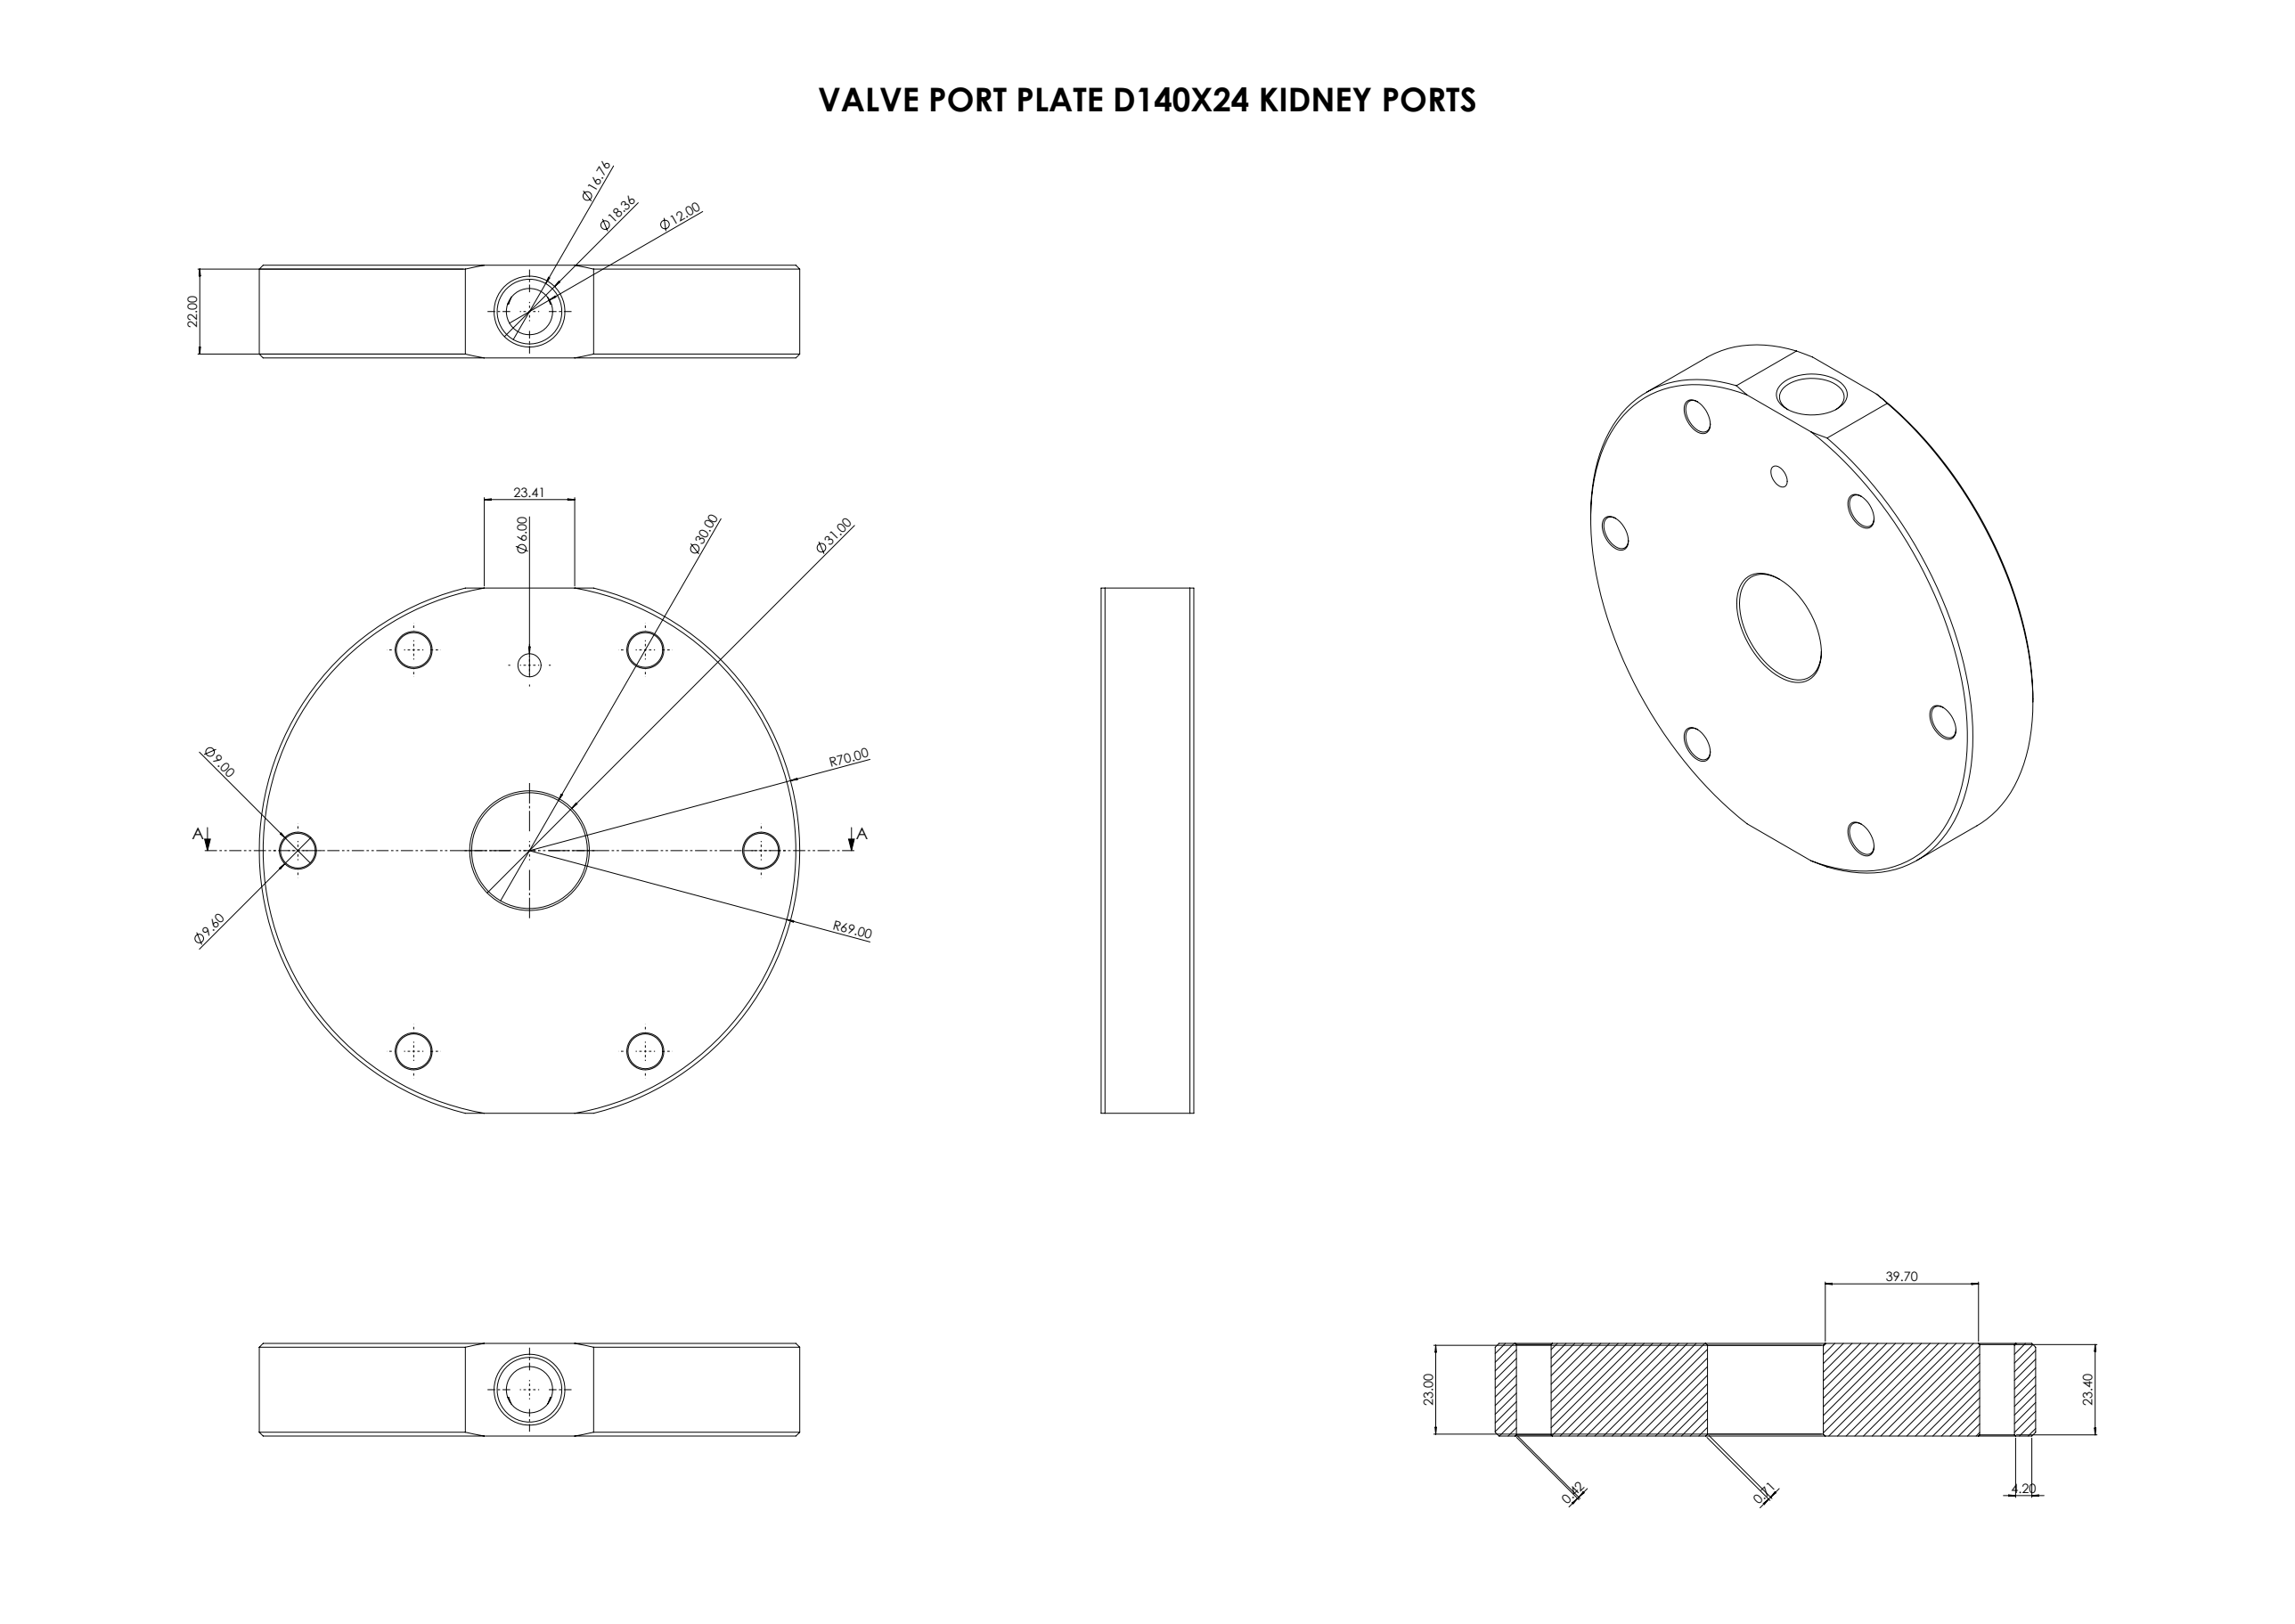
ISO-10303-21;
HEADER;
/* Generated by software containing ST-Developer
 * from STEP Tools, Inc. (www.steptools.com) 
 */

FILE_DESCRIPTION(
/* description */ (''),
/* implementation_level */ '2;1');

FILE_NAME(
/* name */ '02_Valve_Port_Plate_D140x24_Kidney_Ports.step',
/* time_stamp */ '2026-10-23T00:52:27+05:00',
/* author */ (''),
/* organization */ (''),
/* preprocessor_version */ 'ST-DEVELOPER v20.2',
/* originating_system */ 'Autodesk Translation Framework v15.15.0.0',
/* authorisation */ '');

FILE_SCHEMA (('AUTOMOTIVE_DESIGN { 1 0 10303 214 3 1 1 }'));
ENDSEC;

DATA;
#10=MECHANICAL_DESIGN_GEOMETRIC_PRESENTATION_REPRESENTATION('',(#1565),#59204);
#704=B_SPLINE_CURVE_WITH_KNOTS('',3,(#42904,#42905,#42906,#42907,#42908,
#42909,#42910,#42911,#42912,#42913,#42914,#42915,#42916,#42917,#42918,#42919,
#42920,#42921),.UNSPECIFIED.,.F.,.F.,(4,2,2,2,2,2,2,2,4),(0.,0.115474560264442,
0.230949120528883,0.346108891526704,0.461268662524524,0.576428433522344,
0.691588204520164,0.807062764784606,0.922537325049047),.UNSPECIFIED.);
#705=B_SPLINE_CURVE_WITH_KNOTS('',3,(#42922,#42923,#42924,#42925,#42926,
#42927,#42928,#42929,#42930,#42931,#42932,#42933,#42934,#42935,#42936,#42937,
#42938,#42939),.UNSPECIFIED.,.F.,.F.,(4,2,2,2,2,2,2,2,4),(0.922537325049047,
1.03801188531349,1.15348644557793,1.26864621657575,1.38380598757357,1.49896575857139,
1.61412552956921,1.72960008983365,1.84507465009809),.UNSPECIFIED.);
#706=B_SPLINE_CURVE_WITH_KNOTS('',3,(#43005,#43006,#43007,#43008,#43009,
#43010,#43011,#43012,#43013,#43014),.UNSPECIFIED.,.F.,.F.,(4,2,2,2,4),(0.196434861767707,
0.226700589297083,0.453401178594166,0.680088163565136,0.906775148536106),
 .UNSPECIFIED.);
#707=B_SPLINE_CURVE_WITH_KNOTS('',3,(#43021,#43022,#43023,#43024,#43025,
#43026,#43027,#43028,#43029,#43030),.UNSPECIFIED.,.F.,.F.,(4,2,2,2,4),(0.906775148536106,
1.13346213350708,1.36014911847805,1.58684970777513,1.61711543530451),
 .UNSPECIFIED.);
#708=B_SPLINE_CURVE_WITH_KNOTS('',3,(#43034,#43035,#43036,#43037,#43038,
#43039,#43040,#43041,#43042,#43043,#43044,#43045,#43046,#43047),
 .UNSPECIFIED.,.F.,.F.,(4,2,2,2,2,2,4),(2.20122847938268,2.27205851753461,
2.49923948385036,2.72642045016611,2.95360141648186,3.18078238279761,3.25161242094954),
 .UNSPECIFIED.);
#709=B_SPLINE_CURVE_WITH_KNOTS('',3,(#43054,#43055,#43056,#43057,#43058,
#43059),.UNSPECIFIED.,.F.,.F.,(4,2,4),(0.193270693145506,0.23055183180291,
0.366122014076097),.UNSPECIFIED.);
#710=B_SPLINE_CURVE_WITH_KNOTS('',3,(#43067,#43068,#43069,#43070,#43071,
#43072),.UNSPECIFIED.,.F.,.F.,(4,2,4),(1.5242057805381,1.65977596281129,
1.69705710146869),.UNSPECIFIED.);
#711=B_SPLINE_CURVE_WITH_KNOTS('',3,(#43096,#43097,#43098,#43099,#43100,
#43101,#43102,#43103,#43104,#43105),.UNSPECIFIED.,.F.,.F.,(4,2,2,2,4),(2.72032544560832,
2.94701243057929,3.17369941555026,3.40040000484734,3.43066573237672),
 .UNSPECIFIED.);
#712=B_SPLINE_CURVE_WITH_KNOTS('',3,(#43110,#43111,#43112,#43113,#43114,
#43115,#43116,#43117,#43118,#43119),.UNSPECIFIED.,.F.,.F.,(4,2,2,2,4),(2.00998515883992,
2.0402508863693,2.26695147566638,2.49363846063735,2.72032544560832),
 .UNSPECIFIED.);
#713=B_SPLINE_CURVE_WITH_KNOTS('',3,(#43126,#43127,#43128,#43129,#43130,
#43131,#43132,#43133,#43134,#43135,#43136,#43137,#43138,#43139),
 .UNSPECIFIED.,.F.,.F.,(4,2,2,2,2,2,4),(0.383614845938606,0.454444884090536,
0.681625850406286,0.908806816722037,1.13598778303779,1.36316874935354,1.43399878750547),
 .UNSPECIFIED.);
#714=B_SPLINE_CURVE_WITH_KNOTS('',3,(#43147,#43148,#43149,#43150,#43151,
#43152),.UNSPECIFIED.,.F.,.F.,(4,2,4),(2.08359848775971,2.12087962641711,
2.2564498086903),.UNSPECIFIED.);
#715=B_SPLINE_CURVE_WITH_KNOTS('',3,(#43160,#43161,#43162,#43163,#43164,
#43165),.UNSPECIFIED.,.F.,.F.,(4,2,4),(3.4145335751523,3.55010375742549,
3.5873848960829),.UNSPECIFIED.);
#1482=(
BOUNDED_CURVE()
B_SPLINE_CURVE(2,(#42953,#42954,#42955),.UNSPECIFIED.,.F.,.F.)
B_SPLINE_CURVE_WITH_KNOTS((3,3),(0.,0.501003712116266),.UNSPECIFIED.)
CURVE()
GEOMETRIC_REPRESENTATION_ITEM()
RATIONAL_B_SPLINE_CURVE((1.,1.00062409811598,1.))
REPRESENTATION_ITEM('')
);
#1483=(
BOUNDED_CURVE()
B_SPLINE_CURVE(2,(#42958,#42959,#42960),.UNSPECIFIED.,.F.,.F.)
B_SPLINE_CURVE_WITH_KNOTS((3,3),(0.,0.501003712116271),.UNSPECIFIED.)
CURVE()
GEOMETRIC_REPRESENTATION_ITEM()
RATIONAL_B_SPLINE_CURVE((1.,1.00062409811548,1.))
REPRESENTATION_ITEM('')
);
#1484=(
BOUNDED_CURVE()
B_SPLINE_CURVE(2,(#42962,#42963,#42964),.UNSPECIFIED.,.F.,.F.)
B_SPLINE_CURVE_WITH_KNOTS((3,3),(0.,0.501003712116271),.UNSPECIFIED.)
CURVE()
GEOMETRIC_REPRESENTATION_ITEM()
RATIONAL_B_SPLINE_CURVE((1.,1.00062409811548,1.))
REPRESENTATION_ITEM('')
);
#1485=(
BOUNDED_CURVE()
B_SPLINE_CURVE(2,(#42967,#42968,#42969),.UNSPECIFIED.,.F.,.F.)
B_SPLINE_CURVE_WITH_KNOTS((3,3),(0.,0.501003712116266),.UNSPECIFIED.)
CURVE()
GEOMETRIC_REPRESENTATION_ITEM()
RATIONAL_B_SPLINE_CURVE((1.,1.00062409811598,1.))
REPRESENTATION_ITEM('')
);
#1486=(
BOUNDED_CURVE()
B_SPLINE_CURVE(2,(#42982,#42983,#42984),.UNSPECIFIED.,.F.,.F.)
B_SPLINE_CURVE_WITH_KNOTS((3,3),(0.,0.501003712116266),.UNSPECIFIED.)
CURVE()
GEOMETRIC_REPRESENTATION_ITEM()
RATIONAL_B_SPLINE_CURVE((1.,1.00062409811598,1.))
REPRESENTATION_ITEM('')
);
#1487=(
BOUNDED_CURVE()
B_SPLINE_CURVE(2,(#42987,#42988,#42989),.UNSPECIFIED.,.F.,.F.)
B_SPLINE_CURVE_WITH_KNOTS((3,3),(0.,0.501003712116271),.UNSPECIFIED.)
CURVE()
GEOMETRIC_REPRESENTATION_ITEM()
RATIONAL_B_SPLINE_CURVE((1.,1.00062409811541,1.))
REPRESENTATION_ITEM('')
);
#1488=(
BOUNDED_CURVE()
B_SPLINE_CURVE(2,(#42991,#42992,#42993),.UNSPECIFIED.,.F.,.F.)
B_SPLINE_CURVE_WITH_KNOTS((3,3),(0.,0.501003712116271),.UNSPECIFIED.)
CURVE()
GEOMETRIC_REPRESENTATION_ITEM()
RATIONAL_B_SPLINE_CURVE((1.,1.00062409811541,1.))
REPRESENTATION_ITEM('')
);
#1489=(
BOUNDED_CURVE()
B_SPLINE_CURVE(2,(#42996,#42997,#42998),.UNSPECIFIED.,.F.,.F.)
B_SPLINE_CURVE_WITH_KNOTS((3,3),(0.,0.501003712116266),.UNSPECIFIED.)
CURVE()
GEOMETRIC_REPRESENTATION_ITEM()
RATIONAL_B_SPLINE_CURVE((1.,1.00062409811598,1.))
REPRESENTATION_ITEM('')
);
#1490=(
BOUNDED_CURVE()
B_SPLINE_CURVE(2,(#43060,#43061,#43062),.UNSPECIFIED.,.F.,.F.)
B_SPLINE_CURVE_WITH_KNOTS((3,3),(0.,0.0102434961117393),.UNSPECIFIED.)
CURVE()
GEOMETRIC_REPRESENTATION_ITEM()
RATIONAL_B_SPLINE_CURVE((1.,1.01666622123361,1.03305467953702))
REPRESENTATION_ITEM('')
);
#1491=(
BOUNDED_CURVE()
B_SPLINE_CURVE(2,(#43064,#43065,#43066),.UNSPECIFIED.,.F.,.F.)
B_SPLINE_CURVE_WITH_KNOTS((3,3),(1.21900889027555,1.22925238638729),
 .UNSPECIFIED.)
CURVE()
GEOMETRIC_REPRESENTATION_ITEM()
RATIONAL_B_SPLINE_CURVE((1.03305467953703,1.01666622123362,1.))
REPRESENTATION_ITEM('')
);
#1492=(
BOUNDED_CURVE()
B_SPLINE_CURVE(2,(#43153,#43154,#43155),.UNSPECIFIED.,.F.,.F.)
B_SPLINE_CURVE_WITH_KNOTS((3,3),(0.,0.0102434961117392),.UNSPECIFIED.)
CURVE()
GEOMETRIC_REPRESENTATION_ITEM()
RATIONAL_B_SPLINE_CURVE((1.,1.01666622123361,1.03305467953702))
REPRESENTATION_ITEM('')
);
#1493=(
BOUNDED_CURVE()
B_SPLINE_CURVE(2,(#43157,#43158,#43159),.UNSPECIFIED.,.F.,.F.)
B_SPLINE_CURVE_WITH_KNOTS((3,3),(1.21900889027555,1.22925238638729),
 .UNSPECIFIED.)
CURVE()
GEOMETRIC_REPRESENTATION_ITEM()
RATIONAL_B_SPLINE_CURVE((1.03305467953701,1.01666622123361,1.))
REPRESENTATION_ITEM('')
);
#1519=SHAPE_REPRESENTATION_RELATIONSHIP('SRR','None',#59308,#1539);
#1539=ADVANCED_BREP_SHAPE_REPRESENTATION('',(#1586),#59195);
#1565=STYLED_ITEM('',(#59579),#1586);
#1586=MANIFOLD_SOLID_BREP('Valve plate',#22815);
#1694=FACE_BOUND('',#4510,.T.);
#1695=FACE_BOUND('',#4511,.T.);
#1696=FACE_BOUND('',#4512,.T.);
#1697=FACE_BOUND('',#4513,.T.);
#1698=FACE_BOUND('',#4514,.T.);
#1699=FACE_BOUND('',#4515,.T.);
#1700=FACE_BOUND('',#4516,.T.);
#1701=FACE_BOUND('',#4517,.T.);
#1702=FACE_BOUND('',#4520,.T.);
#1703=FACE_BOUND('',#4521,.T.);
#1704=FACE_BOUND('',#4522,.T.);
#1705=FACE_BOUND('',#4523,.T.);
#1706=FACE_BOUND('',#4524,.T.);
#1707=FACE_BOUND('',#4525,.T.);
#1708=FACE_BOUND('',#4526,.T.);
#1709=FACE_BOUND('',#4527,.T.);
#1710=FACE_BOUND('',#4528,.T.);
#1711=FACE_BOUND('',#4548,.T.);
#1712=FACE_BOUND('',#4552,.T.);
#1713=FACE_BOUND('',#4556,.T.);
#1714=FACE_BOUND('',#4564,.T.);
#1715=FACE_BOUND('',#4568,.T.);
#2041=PLANE('',#23872);
#2042=PLANE('',#23884);
#2043=PLANE('',#23932);
#2044=PLANE('',#23938);
#2045=PLANE('',#23945);
#2046=PLANE('',#23950);
#2047=PLANE('',#23965);
#2048=PLANE('',#23969);
#2049=PLANE('',#23977);
#2050=PLANE('',#23983);
#2529=CYLINDRICAL_SURFACE('',#23870,0.45);
#2530=CYLINDRICAL_SURFACE('',#23903,0.45);
#2531=CYLINDRICAL_SURFACE('',#23908,0.45);
#2532=CYLINDRICAL_SURFACE('',#23913,0.45);
#2533=CYLINDRICAL_SURFACE('',#23918,0.45);
#2534=CYLINDRICAL_SURFACE('',#23923,0.45);
#2535=CYLINDRICAL_SURFACE('',#23926,0.3);
#2536=CYLINDRICAL_SURFACE('',#23930,0.8381);
#2537=CYLINDRICAL_SURFACE('',#23936,0.8381);
#2538=CYLINDRICAL_SURFACE('',#23939,0.6);
#2539=CYLINDRICAL_SURFACE('',#23942,0.6);
#2540=CYLINDRICAL_SURFACE('',#23947,2.25);
#2541=CYLINDRICAL_SURFACE('',#23955,7.);
#2542=CYLINDRICAL_SURFACE('',#23958,0.6);
#2543=CYLINDRICAL_SURFACE('',#23961,0.6);
#2544=CYLINDRICAL_SURFACE('',#23966,2.25);
#2545=CYLINDRICAL_SURFACE('',#23972,0.35);
#2546=CYLINDRICAL_SURFACE('',#23974,2.95);
#2547=CYLINDRICAL_SURFACE('',#23976,0.35);
#2548=CYLINDRICAL_SURFACE('',#23978,0.35);
#2549=CYLINDRICAL_SURFACE('',#23980,2.95);
#2550=CYLINDRICAL_SURFACE('',#23982,0.35);
#2551=CYLINDRICAL_SURFACE('',#23987,1.5);
#2552=CYLINDRICAL_SURFACE('',#23993,7.);
#3107=FACE_OUTER_BOUND('',#4507,.T.);
#3108=FACE_OUTER_BOUND('',#4508,.T.);
#3109=FACE_OUTER_BOUND('',#4509,.T.);
#3110=FACE_OUTER_BOUND('',#4518,.T.);
#3111=FACE_OUTER_BOUND('',#4519,.T.);
#3112=FACE_OUTER_BOUND('',#4529,.T.);
#3113=FACE_OUTER_BOUND('',#4530,.T.);
#3114=FACE_OUTER_BOUND('',#4531,.T.);
#3115=FACE_OUTER_BOUND('',#4532,.T.);
#3116=FACE_OUTER_BOUND('',#4533,.T.);
#3117=FACE_OUTER_BOUND('',#4534,.T.);
#3118=FACE_OUTER_BOUND('',#4535,.T.);
#3119=FACE_OUTER_BOUND('',#4536,.T.);
#3120=FACE_OUTER_BOUND('',#4537,.T.);
#3121=FACE_OUTER_BOUND('',#4538,.T.);
#3122=FACE_OUTER_BOUND('',#4539,.T.);
#3123=FACE_OUTER_BOUND('',#4540,.T.);
#3124=FACE_OUTER_BOUND('',#4541,.T.);
#3125=FACE_OUTER_BOUND('',#4542,.T.);
#3126=FACE_OUTER_BOUND('',#4543,.T.);
#3127=FACE_OUTER_BOUND('',#4544,.T.);
#3128=FACE_OUTER_BOUND('',#4545,.T.);
#3129=FACE_OUTER_BOUND('',#4546,.T.);
#3130=FACE_OUTER_BOUND('',#4547,.T.);
#3131=FACE_OUTER_BOUND('',#4549,.T.);
#3132=FACE_OUTER_BOUND('',#4550,.T.);
#3133=FACE_OUTER_BOUND('',#4551,.T.);
#3134=FACE_OUTER_BOUND('',#4553,.T.);
#3135=FACE_OUTER_BOUND('',#4554,.T.);
#3136=FACE_OUTER_BOUND('',#4555,.T.);
#3137=FACE_OUTER_BOUND('',#4557,.T.);
#3138=FACE_OUTER_BOUND('',#4558,.T.);
#3139=FACE_OUTER_BOUND('',#4559,.T.);
#3140=FACE_OUTER_BOUND('',#4560,.T.);
#3141=FACE_OUTER_BOUND('',#4561,.T.);
#3142=FACE_OUTER_BOUND('',#4562,.T.);
#3143=FACE_OUTER_BOUND('',#4563,.T.);
#3144=FACE_OUTER_BOUND('',#4565,.T.);
#3145=FACE_OUTER_BOUND('',#4566,.T.);
#3146=FACE_OUTER_BOUND('',#4567,.T.);
#3147=FACE_OUTER_BOUND('',#4569,.T.);
#3148=FACE_OUTER_BOUND('',#4570,.T.);
#3149=FACE_OUTER_BOUND('',#4571,.T.);
#3150=FACE_OUTER_BOUND('',#4572,.T.);
#3151=FACE_OUTER_BOUND('',#4573,.T.);
#3152=FACE_OUTER_BOUND('',#4574,.T.);
#3153=FACE_OUTER_BOUND('',#4575,.T.);
#3154=FACE_OUTER_BOUND('',#4576,.T.);
#3155=FACE_OUTER_BOUND('',#4577,.T.);
#3156=FACE_OUTER_BOUND('',#4578,.T.);
#3157=FACE_OUTER_BOUND('',#4579,.T.);
#3158=FACE_OUTER_BOUND('',#4580,.T.);
#3159=FACE_OUTER_BOUND('',#4581,.T.);
#3160=FACE_OUTER_BOUND('',#4582,.T.);
#3161=FACE_OUTER_BOUND('',#4583,.T.);
#3162=FACE_OUTER_BOUND('',#4584,.T.);
#4507=EDGE_LOOP('',(#16736,#16737,#16738,#16739));
#4508=EDGE_LOOP('',(#16740,#16741,#16742,#16743));
#4509=EDGE_LOOP('',(#16744,#16745,#16746,#16747));
#4510=EDGE_LOOP('',(#16748));
#4511=EDGE_LOOP('',(#16749));
#4512=EDGE_LOOP('',(#16750));
#4513=EDGE_LOOP('',(#16751));
#4514=EDGE_LOOP('',(#16752));
#4515=EDGE_LOOP('',(#16753));
#4516=EDGE_LOOP('',(#16754));
#4517=EDGE_LOOP('',(#16755));
#4518=EDGE_LOOP('',(#16756,#16757,#16758,#16759));
#4519=EDGE_LOOP('',(#16760,#16761,#16762,#16763));
#4520=EDGE_LOOP('',(#16764));
#4521=EDGE_LOOP('',(#16765));
#4522=EDGE_LOOP('',(#16766));
#4523=EDGE_LOOP('',(#16767,#16768,#16769,#16770));
#4524=EDGE_LOOP('',(#16771,#16772,#16773,#16774));
#4525=EDGE_LOOP('',(#16775));
#4526=EDGE_LOOP('',(#16776));
#4527=EDGE_LOOP('',(#16777));
#4528=EDGE_LOOP('',(#16778));
#4529=EDGE_LOOP('',(#16779,#16780,#16781,#16782));
#4530=EDGE_LOOP('',(#16783,#16784,#16785,#16786));
#4531=EDGE_LOOP('',(#16787,#16788,#16789,#16790));
#4532=EDGE_LOOP('',(#16791,#16792,#16793,#16794));
#4533=EDGE_LOOP('',(#16795,#16796,#16797,#16798));
#4534=EDGE_LOOP('',(#16799,#16800,#16801,#16802));
#4535=EDGE_LOOP('',(#16803,#16804,#16805,#16806));
#4536=EDGE_LOOP('',(#16807,#16808,#16809,#16810));
#4537=EDGE_LOOP('',(#16811,#16812,#16813,#16814));
#4538=EDGE_LOOP('',(#16815,#16816,#16817,#16818));
#4539=EDGE_LOOP('',(#16819,#16820,#16821,#16822));
#4540=EDGE_LOOP('',(#16823,#16824,#16825,#16826));
#4541=EDGE_LOOP('',(#16827,#16828,#16829,#16830));
#4542=EDGE_LOOP('',(#16831,#16832,#16833,#16834));
#4543=EDGE_LOOP('',(#16835,#16836,#16837,#16838));
#4544=EDGE_LOOP('',(#16839,#16840,#16841,#16842,#16843));
#4545=EDGE_LOOP('',(#16844,#16845,#16846,#16847));
#4546=EDGE_LOOP('',(#16848,#16849,#16850,#16851));
#4547=EDGE_LOOP('',(#16852,#16853,#16854,#16855,#16856,#16857,#16858,#16859));
#4548=EDGE_LOOP('',(#16860));
#4549=EDGE_LOOP('',(#16861,#16862,#16863,#16864));
#4550=EDGE_LOOP('',(#16865,#16866,#16867,#16868));
#4551=EDGE_LOOP('',(#16869,#16870,#16871,#16872,#16873,#16874,#16875,#16876));
#4552=EDGE_LOOP('',(#16877));
#4553=EDGE_LOOP('',(#16878,#16879,#16880,#16881,#16882,#16883,#16884,#16885));
#4554=EDGE_LOOP('',(#16886,#16887,#16888));
#4555=EDGE_LOOP('',(#16889));
#4556=EDGE_LOOP('',(#16890));
#4557=EDGE_LOOP('',(#16891,#16892,#16893,#16894,#16895,#16896,#16897,#16898,
#16899));
#4558=EDGE_LOOP('',(#16900,#16901,#16902,#16903,#16904,#16905,#16906,#16907));
#4559=EDGE_LOOP('',(#16908,#16909,#16910,#16911,#16912));
#4560=EDGE_LOOP('',(#16913,#16914,#16915,#16916));
#4561=EDGE_LOOP('',(#16917,#16918,#16919,#16920));
#4562=EDGE_LOOP('',(#16921,#16922,#16923,#16924));
#4563=EDGE_LOOP('',(#16925,#16926,#16927,#16928,#16929,#16930,#16931,#16932));
#4564=EDGE_LOOP('',(#16933,#16934));
#4565=EDGE_LOOP('',(#16935,#16936,#16937));
#4566=EDGE_LOOP('',(#16938,#16939,#16940,#16941,#16942,#16943,#16944,#16945,
#16946));
#4567=EDGE_LOOP('',(#16947));
#4568=EDGE_LOOP('',(#16948));
#4569=EDGE_LOOP('',(#16949,#16950,#16951,#16952,#16953,#16954,#16955,#16956));
#4570=EDGE_LOOP('',(#16957,#16958,#16959,#16960,#16961));
#4571=EDGE_LOOP('',(#16962,#16963,#16964,#16965));
#4572=EDGE_LOOP('',(#16966,#16967,#16968,#16969,#16970,#16971,#16972));
#4573=EDGE_LOOP('',(#16973,#16974,#16975,#16976));
#4574=EDGE_LOOP('',(#16977,#16978,#16979,#16980,#16981));
#4575=EDGE_LOOP('',(#16982,#16983,#16984,#16985));
#4576=EDGE_LOOP('',(#16986,#16987,#16988,#16989,#16990,#16991,#16992));
#4577=EDGE_LOOP('',(#16993,#16994,#16995,#16996));
#4578=EDGE_LOOP('',(#16997,#16998,#16999,#17000,#17001));
#4579=EDGE_LOOP('',(#17002,#17003,#17004,#17005,#17006));
#4580=EDGE_LOOP('',(#17007,#17008,#17009,#17010,#17011,#17012));
#4581=EDGE_LOOP('',(#17013,#17014,#17015,#17016,#17017));
#4582=EDGE_LOOP('',(#17018,#17019,#17020,#17021));
#4583=EDGE_LOOP('',(#17022,#17023,#17024,#17025));
#4584=EDGE_LOOP('',(#17026,#17027,#17028,#17029));
#5973=LINE('',#42781,#7406);
#5974=LINE('',#42786,#7407);
#5975=LINE('',#42790,#7408);
#5976=LINE('',#42794,#7409);
#5977=LINE('',#42813,#7410);
#5978=LINE('',#42817,#7411);
#5979=LINE('',#42821,#7412);
#5980=LINE('',#42853,#7413);
#5981=LINE('',#42858,#7414);
#5982=LINE('',#42860,#7415);
#5983=LINE('',#42863,#7416);
#5984=LINE('',#42868,#7417);
#5985=LINE('',#42870,#7418);
#5986=LINE('',#42873,#7419);
#5987=LINE('',#42878,#7420);
#5988=LINE('',#42880,#7421);
#5989=LINE('',#42883,#7422);
#5990=LINE('',#42888,#7423);
#5991=LINE('',#42890,#7424);
#5992=LINE('',#42893,#7425);
#5993=LINE('',#42898,#7426);
#5994=LINE('',#42900,#7427);
#5995=LINE('',#42940,#7428);
#5996=LINE('',#42945,#7429);
#5997=LINE('',#42950,#7430);
#5998=LINE('',#42957,#7431);
#5999=LINE('',#42966,#7432);
#6000=LINE('',#42974,#7433);
#6001=LINE('',#42978,#7434);
#6002=LINE('',#42986,#7435);
#6003=LINE('',#42995,#7436);
#6004=LINE('',#43003,#7437);
#6005=LINE('',#43016,#7438);
#6006=LINE('',#43020,#7439);
#6007=LINE('',#43074,#7440);
#6008=LINE('',#43078,#7441);
#6009=LINE('',#43080,#7442);
#6010=LINE('',#43094,#7443);
#6011=LINE('',#43107,#7444);
#6012=LINE('',#43121,#7445);
#6013=LINE('',#43145,#7446);
#6014=LINE('',#43170,#7447);
#6015=LINE('',#43172,#7448);
#6016=LINE('',#43180,#7449);
#6017=LINE('',#43184,#7450);
#6018=LINE('',#43189,#7451);
#6019=LINE('',#43193,#7452);
#6020=LINE('',#43198,#7453);
#6021=LINE('',#43207,#7454);
#6022=LINE('',#43209,#7455);
#7406=VECTOR('',#27247,0.465);
#7407=VECTOR('',#27254,0.45);
#7408=VECTOR('',#27257,1.);
#7409=VECTOR('',#27260,1.);
#7410=VECTOR('',#27281,0.465);
#7411=VECTOR('',#27284,1.);
#7412=VECTOR('',#27287,1.);
#7413=VECTOR('',#27320,0.465);
#7414=VECTOR('',#27327,0.45);
#7415=VECTOR('',#27330,0.465);
#7416=VECTOR('',#27333,0.465);
#7417=VECTOR('',#27340,0.45);
#7418=VECTOR('',#27343,0.465);
#7419=VECTOR('',#27346,0.465);
#7420=VECTOR('',#27353,0.45);
#7421=VECTOR('',#27356,0.465);
#7422=VECTOR('',#27359,0.465);
#7423=VECTOR('',#27366,0.45);
#7424=VECTOR('',#27369,0.465);
#7425=VECTOR('',#27372,0.465);
#7426=VECTOR('',#27379,0.45);
#7427=VECTOR('',#27382,0.465);
#7428=VECTOR('',#27385,0.3);
#7429=VECTOR('',#27390,0.8781);
#7430=VECTOR('',#27397,0.8381);
#7431=VECTOR('',#27400,1.);
#7432=VECTOR('',#27401,1.);
#7433=VECTOR('',#27406,0.8781);
#7434=VECTOR('',#27411,0.8381);
#7435=VECTOR('',#27416,1.);
#7436=VECTOR('',#27417,1.);
#7437=VECTOR('',#27422,0.6);
#7438=VECTOR('',#27423,1.);
#7439=VECTOR('',#27426,1.);
#7440=VECTOR('',#27437,0.6);
#7441=VECTOR('',#27442,1.);
#7442=VECTOR('',#27443,1.);
#7443=VECTOR('',#27464,1.);
#7444=VECTOR('',#27465,0.6);
#7445=VECTOR('',#27468,1.);
#7446=VECTOR('',#27479,0.3);
#7447=VECTOR('',#27486,1.);
#7448=VECTOR('',#27487,1.);
#7449=VECTOR('',#27498,1.);
#7450=VECTOR('',#27505,1.);
#7451=VECTOR('',#27512,1.);
#7452=VECTOR('',#27519,1.);
#7453=VECTOR('',#27526,1.525);
#7454=VECTOR('',#27537,1.5);
#7455=VECTOR('',#27540,1.525);
#8745=CIRCLE('',#23868,0.48);
#8746=CIRCLE('',#23869,0.45);
#8747=CIRCLE('',#23871,0.45);
#8748=CIRCLE('',#23873,6.9);
#8749=CIRCLE('',#23874,6.9);
#8750=CIRCLE('',#23875,0.48);
#8751=CIRCLE('',#23876,0.48);
#8752=CIRCLE('',#23877,0.48);
#8753=CIRCLE('',#23878,1.55);
#8754=CIRCLE('',#23879,0.3);
#8755=CIRCLE('',#23880,0.48);
#8756=CIRCLE('',#23881,0.48);
#8757=CIRCLE('',#23883,0.48);
#8758=CIRCLE('',#23885,6.9);
#8759=CIRCLE('',#23886,6.9);
#8760=CIRCLE('',#23887,0.48);
#8761=CIRCLE('',#23888,0.48);
#8762=CIRCLE('',#23889,0.48);
#8763=CIRCLE('',#23890,2.25);
#8764=CIRCLE('',#23891,0.35);
#8765=CIRCLE('',#23892,2.95);
#8766=CIRCLE('',#23893,0.35);
#8767=CIRCLE('',#23894,2.25);
#8768=CIRCLE('',#23895,0.35);
#8769=CIRCLE('',#23896,2.95);
#8770=CIRCLE('',#23897,0.35);
#8771=CIRCLE('',#23898,1.55);
#8772=CIRCLE('',#23899,0.48);
#8773=CIRCLE('',#23900,0.48);
#8774=CIRCLE('',#23902,0.45);
#8775=CIRCLE('',#23904,0.45);
#8776=CIRCLE('',#23907,0.45);
#8777=CIRCLE('',#23909,0.45);
#8778=CIRCLE('',#23912,0.45);
#8779=CIRCLE('',#23914,0.45);
#8780=CIRCLE('',#23917,0.45);
#8781=CIRCLE('',#23919,0.45);
#8782=CIRCLE('',#23922,0.45);
#8783=CIRCLE('',#23924,0.45);
#8784=CIRCLE('',#23928,0.9181);
#8785=CIRCLE('',#23929,0.8381);
#8786=CIRCLE('',#23931,0.8381);
#8787=CIRCLE('',#23934,0.9181);
#8788=CIRCLE('',#23935,0.8381);
#8789=CIRCLE('',#23937,0.8381);
#8790=CIRCLE('',#23940,0.6);
#8791=CIRCLE('',#23941,0.6);
#8792=CIRCLE('',#23943,0.6);
#8793=CIRCLE('',#23944,0.6);
#8794=CIRCLE('',#23948,2.25);
#8795=CIRCLE('',#23949,2.25);
#8796=CIRCLE('',#23951,2.95);
#8797=CIRCLE('',#23952,0.35);
#8798=CIRCLE('',#23954,7.);
#8799=CIRCLE('',#23956,7.);
#8800=CIRCLE('',#23959,0.6);
#8801=CIRCLE('',#23960,0.6);
#8802=CIRCLE('',#23962,0.6);
#8803=CIRCLE('',#23963,0.6);
#8804=CIRCLE('',#23967,2.25);
#8805=CIRCLE('',#23968,2.25);
#8806=CIRCLE('',#23970,2.95);
#8807=CIRCLE('',#23971,0.35);
#8808=CIRCLE('',#23973,0.35);
#8809=CIRCLE('',#23975,2.95);
#8810=CIRCLE('',#23979,0.35);
#8811=CIRCLE('',#23981,2.95);
#8812=CIRCLE('',#23985,1.5);
#8813=CIRCLE('',#23986,1.5);
#8814=CIRCLE('',#23988,1.5);
#8815=CIRCLE('',#23989,1.5);
#8816=CIRCLE('',#23992,7.);
#8817=CIRCLE('',#23994,7.);
#9846=VERTEX_POINT('',#42778);
#9847=VERTEX_POINT('',#42780);
#9848=VERTEX_POINT('',#42784);
#9849=VERTEX_POINT('',#42788);
#9850=VERTEX_POINT('',#42789);
#9851=VERTEX_POINT('',#42791);
#9852=VERTEX_POINT('',#42793);
#9853=VERTEX_POINT('',#42796);
#9854=VERTEX_POINT('',#42798);
#9855=VERTEX_POINT('',#42800);
#9856=VERTEX_POINT('',#42802);
#9857=VERTEX_POINT('',#42804);
#9858=VERTEX_POINT('',#42806);
#9859=VERTEX_POINT('',#42808);
#9860=VERTEX_POINT('',#42811);
#9861=VERTEX_POINT('',#42815);
#9862=VERTEX_POINT('',#42816);
#9863=VERTEX_POINT('',#42818);
#9864=VERTEX_POINT('',#42820);
#9865=VERTEX_POINT('',#42823);
#9866=VERTEX_POINT('',#42825);
#9867=VERTEX_POINT('',#42827);
#9868=VERTEX_POINT('',#42829);
#9869=VERTEX_POINT('',#42830);
#9870=VERTEX_POINT('',#42832);
#9871=VERTEX_POINT('',#42834);
#9872=VERTEX_POINT('',#42837);
#9873=VERTEX_POINT('',#42838);
#9874=VERTEX_POINT('',#42840);
#9875=VERTEX_POINT('',#42842);
#9876=VERTEX_POINT('',#42845);
#9877=VERTEX_POINT('',#42847);
#9878=VERTEX_POINT('',#42849);
#9879=VERTEX_POINT('',#42852);
#9880=VERTEX_POINT('',#42856);
#9881=VERTEX_POINT('',#42862);
#9882=VERTEX_POINT('',#42866);
#9883=VERTEX_POINT('',#42872);
#9884=VERTEX_POINT('',#42876);
#9885=VERTEX_POINT('',#42882);
#9886=VERTEX_POINT('',#42886);
#9887=VERTEX_POINT('',#42892);
#9888=VERTEX_POINT('',#42896);
#9889=VERTEX_POINT('',#42902);
#9890=VERTEX_POINT('',#42903);
#9891=VERTEX_POINT('',#42942);
#9892=VERTEX_POINT('',#42944);
#9893=VERTEX_POINT('',#42948);
#9894=VERTEX_POINT('',#42952);
#9895=VERTEX_POINT('',#42956);
#9896=VERTEX_POINT('',#42961);
#9897=VERTEX_POINT('',#42965);
#9898=VERTEX_POINT('',#42971);
#9899=VERTEX_POINT('',#42973);
#9900=VERTEX_POINT('',#42977);
#9901=VERTEX_POINT('',#42981);
#9902=VERTEX_POINT('',#42985);
#9903=VERTEX_POINT('',#42990);
#9904=VERTEX_POINT('',#42994);
#9905=VERTEX_POINT('',#43000);
#9906=VERTEX_POINT('',#43002);
#9907=VERTEX_POINT('',#43004);
#9908=VERTEX_POINT('',#43015);
#9909=VERTEX_POINT('',#43017);
#9910=VERTEX_POINT('',#43019);
#9911=VERTEX_POINT('',#43032);
#9912=VERTEX_POINT('',#43033);
#9913=VERTEX_POINT('',#43048);
#9914=VERTEX_POINT('',#43053);
#9915=VERTEX_POINT('',#43063);
#9916=VERTEX_POINT('',#43073);
#9917=VERTEX_POINT('',#43076);
#9918=VERTEX_POINT('',#43079);
#9919=VERTEX_POINT('',#43083);
#9920=VERTEX_POINT('',#43092);
#9921=VERTEX_POINT('',#43093);
#9922=VERTEX_POINT('',#43095);
#9923=VERTEX_POINT('',#43106);
#9924=VERTEX_POINT('',#43109);
#9925=VERTEX_POINT('',#43120);
#9926=VERTEX_POINT('',#43124);
#9927=VERTEX_POINT('',#43125);
#9928=VERTEX_POINT('',#43140);
#9929=VERTEX_POINT('',#43144);
#9930=VERTEX_POINT('',#43146);
#9931=VERTEX_POINT('',#43156);
#9932=VERTEX_POINT('',#43168);
#9933=VERTEX_POINT('',#43171);
#9934=VERTEX_POINT('',#43175);
#9935=VERTEX_POINT('',#43179);
#9936=VERTEX_POINT('',#43188);
#9937=VERTEX_POINT('',#43197);
#9938=VERTEX_POINT('',#43199);
#9939=VERTEX_POINT('',#43203);
#9940=VERTEX_POINT('',#43204);
#12372=EDGE_CURVE('',#9846,#9846,#8745,.T.);
#12373=EDGE_CURVE('',#9846,#9847,#5973,.T.);
#12374=EDGE_CURVE('',#9847,#9847,#8746,.T.);
#12375=EDGE_CURVE('',#9848,#9848,#8747,.T.);
#12376=EDGE_CURVE('',#9848,#9847,#5974,.T.);
#12377=EDGE_CURVE('',#9849,#9850,#5975,.T.);
#12378=EDGE_CURVE('',#9850,#9851,#8748,.T.);
#12379=EDGE_CURVE('',#9851,#9852,#5976,.T.);
#12380=EDGE_CURVE('',#9852,#9849,#8749,.T.);
#12381=EDGE_CURVE('',#9853,#9853,#8750,.T.);
#12382=EDGE_CURVE('',#9854,#9854,#8751,.T.);
#12383=EDGE_CURVE('',#9855,#9855,#8752,.T.);
#12384=EDGE_CURVE('',#9856,#9856,#8753,.T.);
#12385=EDGE_CURVE('',#9857,#9857,#8754,.T.);
#12386=EDGE_CURVE('',#9858,#9858,#8755,.T.);
#12387=EDGE_CURVE('',#9859,#9859,#8756,.T.);
#12388=EDGE_CURVE('',#9860,#9860,#8757,.T.);
#12389=EDGE_CURVE('',#9860,#9848,#5977,.T.);
#12390=EDGE_CURVE('',#9861,#9862,#5978,.T.);
#12391=EDGE_CURVE('',#9863,#9862,#8758,.T.);
#12392=EDGE_CURVE('',#9863,#9864,#5979,.T.);
#12393=EDGE_CURVE('',#9861,#9864,#8759,.T.);
#12394=EDGE_CURVE('',#9865,#9865,#8760,.T.);
#12395=EDGE_CURVE('',#9866,#9866,#8761,.T.);
#12396=EDGE_CURVE('',#9867,#9867,#8762,.T.);
#12397=EDGE_CURVE('',#9868,#9869,#8763,.T.);
#12398=EDGE_CURVE('',#9869,#9870,#8764,.T.);
#12399=EDGE_CURVE('',#9870,#9871,#8765,.T.);
#12400=EDGE_CURVE('',#9871,#9868,#8766,.T.);
#12401=EDGE_CURVE('',#9872,#9873,#8767,.T.);
#12402=EDGE_CURVE('',#9873,#9874,#8768,.T.);
#12403=EDGE_CURVE('',#9874,#9875,#8769,.T.);
#12404=EDGE_CURVE('',#9875,#9872,#8770,.T.);
#12405=EDGE_CURVE('',#9876,#9876,#8771,.T.);
#12406=EDGE_CURVE('',#9877,#9877,#8772,.T.);
#12407=EDGE_CURVE('',#9878,#9878,#8773,.T.);
#12408=EDGE_CURVE('',#9853,#9879,#5980,.T.);
#12409=EDGE_CURVE('',#9879,#9879,#8774,.T.);
#12410=EDGE_CURVE('',#9880,#9880,#8775,.T.);
#12411=EDGE_CURVE('',#9880,#9879,#5981,.T.);
#12412=EDGE_CURVE('',#9865,#9880,#5982,.T.);
#12413=EDGE_CURVE('',#9859,#9881,#5983,.T.);
#12414=EDGE_CURVE('',#9881,#9881,#8776,.T.);
#12415=EDGE_CURVE('',#9882,#9882,#8777,.T.);
#12416=EDGE_CURVE('',#9882,#9881,#5984,.T.);
#12417=EDGE_CURVE('',#9878,#9882,#5985,.T.);
#12418=EDGE_CURVE('',#9854,#9883,#5986,.T.);
#12419=EDGE_CURVE('',#9883,#9883,#8778,.T.);
#12420=EDGE_CURVE('',#9884,#9884,#8779,.T.);
#12421=EDGE_CURVE('',#9884,#9883,#5987,.T.);
#12422=EDGE_CURVE('',#9866,#9884,#5988,.T.);
#12423=EDGE_CURVE('',#9858,#9885,#5989,.T.);
#12424=EDGE_CURVE('',#9885,#9885,#8780,.T.);
#12425=EDGE_CURVE('',#9886,#9886,#8781,.T.);
#12426=EDGE_CURVE('',#9886,#9885,#5990,.T.);
#12427=EDGE_CURVE('',#9877,#9886,#5991,.T.);
#12428=EDGE_CURVE('',#9855,#9887,#5992,.T.);
#12429=EDGE_CURVE('',#9887,#9887,#8782,.T.);
#12430=EDGE_CURVE('',#9888,#9888,#8783,.T.);
#12431=EDGE_CURVE('',#9888,#9887,#5993,.T.);
#12432=EDGE_CURVE('',#9867,#9888,#5994,.T.);
#12433=EDGE_CURVE('',#9889,#9890,#704,.T.);
#12434=EDGE_CURVE('',#9890,#9889,#705,.T.);
#12435=EDGE_CURVE('',#9890,#9857,#5995,.T.);
#12436=EDGE_CURVE('',#9891,#9891,#8784,.T.);
#12437=EDGE_CURVE('',#9891,#9892,#5996,.T.);
#12438=EDGE_CURVE('',#9892,#9892,#8785,.T.);
#12439=EDGE_CURVE('',#9893,#9893,#8786,.T.);
#12440=EDGE_CURVE('',#9893,#9892,#5997,.T.);
#12441=EDGE_CURVE('',#9894,#9851,#1482,.T.);
#12442=EDGE_CURVE('',#9895,#9894,#5998,.T.);
#12443=EDGE_CURVE('',#9864,#9895,#1483,.T.);
#12444=EDGE_CURVE('',#9896,#9863,#1484,.T.);
#12445=EDGE_CURVE('',#9897,#9896,#5999,.T.);
#12446=EDGE_CURVE('',#9852,#9897,#1485,.T.);
#12447=EDGE_CURVE('',#9898,#9898,#8787,.T.);
#12448=EDGE_CURVE('',#9898,#9899,#6000,.T.);
#12449=EDGE_CURVE('',#9899,#9899,#8788,.T.);
#12450=EDGE_CURVE('',#9899,#9900,#6001,.T.);
#12451=EDGE_CURVE('',#9900,#9900,#8789,.T.);
#12452=EDGE_CURVE('',#9901,#9849,#1486,.T.);
#12453=EDGE_CURVE('',#9902,#9901,#6002,.T.);
#12454=EDGE_CURVE('',#9862,#9902,#1487,.T.);
#12455=EDGE_CURVE('',#9903,#9861,#1488,.T.);
#12456=EDGE_CURVE('',#9904,#9903,#6003,.T.);
#12457=EDGE_CURVE('',#9850,#9904,#1489,.T.);
#12458=EDGE_CURVE('',#9905,#9905,#8790,.T.);
#12459=EDGE_CURVE('',#9905,#9906,#6004,.T.);
#12460=EDGE_CURVE('',#9907,#9906,#706,.T.);
#12461=EDGE_CURVE('',#9908,#9907,#6005,.T.);
#12462=EDGE_CURVE('',#9908,#9909,#8791,.T.);
#12463=EDGE_CURVE('',#9910,#9909,#6006,.T.);
#12464=EDGE_CURVE('',#9906,#9910,#707,.T.);
#12465=EDGE_CURVE('',#9911,#9912,#708,.T.);
#12466=EDGE_CURVE('',#9911,#9913,#8792,.T.);
#12467=EDGE_CURVE('',#9913,#9912,#8793,.T.);
#12468=EDGE_CURVE('',#9914,#9911,#709,.T.);
#12469=EDGE_CURVE('',#9909,#9914,#1490,.T.);
#12470=EDGE_CURVE('',#9915,#9908,#1491,.T.);
#12471=EDGE_CURVE('',#9912,#9915,#710,.T.);
#12472=EDGE_CURVE('',#9913,#9916,#6007,.T.);
#12473=EDGE_CURVE('',#9915,#9917,#8794,.T.);
#12474=EDGE_CURVE('',#9873,#9917,#6008,.T.);
#12475=EDGE_CURVE('',#9872,#9918,#6009,.T.);
#12476=EDGE_CURVE('',#9918,#9914,#8795,.T.);
#12477=EDGE_CURVE('',#9919,#9907,#8796,.T.);
#12478=EDGE_CURVE('',#9917,#9919,#8797,.T.);
#12479=EDGE_CURVE('',#9896,#9902,#8798,.T.);
#12480=EDGE_CURVE('',#9897,#9901,#8799,.T.);
#12481=EDGE_CURVE('',#9920,#9921,#6010,.T.);
#12482=EDGE_CURVE('',#9922,#9920,#711,.T.);
#12483=EDGE_CURVE('',#9922,#9923,#6011,.T.);
#12484=EDGE_CURVE('',#9923,#9923,#8800,.T.);
#12485=EDGE_CURVE('',#9924,#9922,#712,.T.);
#12486=EDGE_CURVE('',#9925,#9924,#6012,.T.);
#12487=EDGE_CURVE('',#9921,#9925,#8801,.T.);
#12488=EDGE_CURVE('',#9926,#9927,#713,.T.);
#12489=EDGE_CURVE('',#9928,#9926,#8802,.T.);
#12490=EDGE_CURVE('',#9927,#9928,#8803,.T.);
#12491=EDGE_CURVE('',#9929,#9928,#6013,.T.);
#12492=EDGE_CURVE('',#9930,#9926,#714,.T.);
#12493=EDGE_CURVE('',#9921,#9930,#1492,.T.);
#12494=EDGE_CURVE('',#9931,#9925,#1493,.T.);
#12495=EDGE_CURVE('',#9927,#9931,#715,.T.);
#12496=EDGE_CURVE('',#9931,#9932,#8804,.T.);
#12497=EDGE_CURVE('',#9869,#9932,#6014,.T.);
#12498=EDGE_CURVE('',#9868,#9933,#6015,.T.);
#12499=EDGE_CURVE('',#9933,#9930,#8805,.T.);
#12500=EDGE_CURVE('',#9934,#9924,#8806,.T.);
#12501=EDGE_CURVE('',#9932,#9934,#8807,.T.);
#12502=EDGE_CURVE('',#9871,#9935,#6016,.T.);
#12503=EDGE_CURVE('',#9935,#9933,#8808,.T.);
#12504=EDGE_CURVE('',#9920,#9935,#8809,.T.);
#12505=EDGE_CURVE('',#9870,#9934,#6017,.T.);
#12506=EDGE_CURVE('',#9875,#9936,#6018,.T.);
#12507=EDGE_CURVE('',#9936,#9918,#8810,.T.);
#12508=EDGE_CURVE('',#9910,#9936,#8811,.T.);
#12509=EDGE_CURVE('',#9874,#9919,#6019,.T.);
#12510=EDGE_CURVE('',#9876,#9937,#6020,.T.);
#12511=EDGE_CURVE('',#9937,#9938,#8812,.T.);
#12512=EDGE_CURVE('',#9938,#9937,#8813,.T.);
#12513=EDGE_CURVE('',#9939,#9940,#8814,.T.);
#12514=EDGE_CURVE('',#9940,#9939,#8815,.T.);
#12515=EDGE_CURVE('',#9940,#9938,#6021,.T.);
#12516=EDGE_CURVE('',#9939,#9856,#6022,.T.);
#12517=EDGE_CURVE('',#9903,#9895,#8816,.T.);
#12518=EDGE_CURVE('',#9904,#9894,#8817,.T.);
#16736=ORIENTED_EDGE('',*,*,#12372,.T.);
#16737=ORIENTED_EDGE('',*,*,#12373,.T.);
#16738=ORIENTED_EDGE('',*,*,#12374,.T.);
#16739=ORIENTED_EDGE('',*,*,#12373,.F.);
#16740=ORIENTED_EDGE('',*,*,#12375,.F.);
#16741=ORIENTED_EDGE('',*,*,#12376,.T.);
#16742=ORIENTED_EDGE('',*,*,#12374,.F.);
#16743=ORIENTED_EDGE('',*,*,#12376,.F.);
#16744=ORIENTED_EDGE('',*,*,#12377,.T.);
#16745=ORIENTED_EDGE('',*,*,#12378,.T.);
#16746=ORIENTED_EDGE('',*,*,#12379,.T.);
#16747=ORIENTED_EDGE('',*,*,#12380,.T.);
#16748=ORIENTED_EDGE('',*,*,#12381,.F.);
#16749=ORIENTED_EDGE('',*,*,#12382,.F.);
#16750=ORIENTED_EDGE('',*,*,#12383,.F.);
#16751=ORIENTED_EDGE('',*,*,#12384,.F.);
#16752=ORIENTED_EDGE('',*,*,#12385,.T.);
#16753=ORIENTED_EDGE('',*,*,#12386,.F.);
#16754=ORIENTED_EDGE('',*,*,#12387,.F.);
#16755=ORIENTED_EDGE('',*,*,#12372,.F.);
#16756=ORIENTED_EDGE('',*,*,#12388,.T.);
#16757=ORIENTED_EDGE('',*,*,#12389,.T.);
#16758=ORIENTED_EDGE('',*,*,#12375,.T.);
#16759=ORIENTED_EDGE('',*,*,#12389,.F.);
#16760=ORIENTED_EDGE('',*,*,#12390,.T.);
#16761=ORIENTED_EDGE('',*,*,#12391,.F.);
#16762=ORIENTED_EDGE('',*,*,#12392,.T.);
#16763=ORIENTED_EDGE('',*,*,#12393,.F.);
#16764=ORIENTED_EDGE('',*,*,#12394,.F.);
#16765=ORIENTED_EDGE('',*,*,#12395,.F.);
#16766=ORIENTED_EDGE('',*,*,#12396,.F.);
#16767=ORIENTED_EDGE('',*,*,#12397,.T.);
#16768=ORIENTED_EDGE('',*,*,#12398,.T.);
#16769=ORIENTED_EDGE('',*,*,#12399,.T.);
#16770=ORIENTED_EDGE('',*,*,#12400,.T.);
#16771=ORIENTED_EDGE('',*,*,#12401,.T.);
#16772=ORIENTED_EDGE('',*,*,#12402,.T.);
#16773=ORIENTED_EDGE('',*,*,#12403,.T.);
#16774=ORIENTED_EDGE('',*,*,#12404,.T.);
#16775=ORIENTED_EDGE('',*,*,#12405,.F.);
#16776=ORIENTED_EDGE('',*,*,#12406,.F.);
#16777=ORIENTED_EDGE('',*,*,#12407,.F.);
#16778=ORIENTED_EDGE('',*,*,#12388,.F.);
#16779=ORIENTED_EDGE('',*,*,#12381,.T.);
#16780=ORIENTED_EDGE('',*,*,#12408,.T.);
#16781=ORIENTED_EDGE('',*,*,#12409,.T.);
#16782=ORIENTED_EDGE('',*,*,#12408,.F.);
#16783=ORIENTED_EDGE('',*,*,#12410,.F.);
#16784=ORIENTED_EDGE('',*,*,#12411,.T.);
#16785=ORIENTED_EDGE('',*,*,#12409,.F.);
#16786=ORIENTED_EDGE('',*,*,#12411,.F.);
#16787=ORIENTED_EDGE('',*,*,#12394,.T.);
#16788=ORIENTED_EDGE('',*,*,#12412,.T.);
#16789=ORIENTED_EDGE('',*,*,#12410,.T.);
#16790=ORIENTED_EDGE('',*,*,#12412,.F.);
#16791=ORIENTED_EDGE('',*,*,#12387,.T.);
#16792=ORIENTED_EDGE('',*,*,#12413,.T.);
#16793=ORIENTED_EDGE('',*,*,#12414,.T.);
#16794=ORIENTED_EDGE('',*,*,#12413,.F.);
#16795=ORIENTED_EDGE('',*,*,#12415,.F.);
#16796=ORIENTED_EDGE('',*,*,#12416,.T.);
#16797=ORIENTED_EDGE('',*,*,#12414,.F.);
#16798=ORIENTED_EDGE('',*,*,#12416,.F.);
#16799=ORIENTED_EDGE('',*,*,#12407,.T.);
#16800=ORIENTED_EDGE('',*,*,#12417,.T.);
#16801=ORIENTED_EDGE('',*,*,#12415,.T.);
#16802=ORIENTED_EDGE('',*,*,#12417,.F.);
#16803=ORIENTED_EDGE('',*,*,#12382,.T.);
#16804=ORIENTED_EDGE('',*,*,#12418,.T.);
#16805=ORIENTED_EDGE('',*,*,#12419,.T.);
#16806=ORIENTED_EDGE('',*,*,#12418,.F.);
#16807=ORIENTED_EDGE('',*,*,#12420,.F.);
#16808=ORIENTED_EDGE('',*,*,#12421,.T.);
#16809=ORIENTED_EDGE('',*,*,#12419,.F.);
#16810=ORIENTED_EDGE('',*,*,#12421,.F.);
#16811=ORIENTED_EDGE('',*,*,#12395,.T.);
#16812=ORIENTED_EDGE('',*,*,#12422,.T.);
#16813=ORIENTED_EDGE('',*,*,#12420,.T.);
#16814=ORIENTED_EDGE('',*,*,#12422,.F.);
#16815=ORIENTED_EDGE('',*,*,#12386,.T.);
#16816=ORIENTED_EDGE('',*,*,#12423,.T.);
#16817=ORIENTED_EDGE('',*,*,#12424,.T.);
#16818=ORIENTED_EDGE('',*,*,#12423,.F.);
#16819=ORIENTED_EDGE('',*,*,#12425,.F.);
#16820=ORIENTED_EDGE('',*,*,#12426,.T.);
#16821=ORIENTED_EDGE('',*,*,#12424,.F.);
#16822=ORIENTED_EDGE('',*,*,#12426,.F.);
#16823=ORIENTED_EDGE('',*,*,#12406,.T.);
#16824=ORIENTED_EDGE('',*,*,#12427,.T.);
#16825=ORIENTED_EDGE('',*,*,#12425,.T.);
#16826=ORIENTED_EDGE('',*,*,#12427,.F.);
#16827=ORIENTED_EDGE('',*,*,#12383,.T.);
#16828=ORIENTED_EDGE('',*,*,#12428,.T.);
#16829=ORIENTED_EDGE('',*,*,#12429,.T.);
#16830=ORIENTED_EDGE('',*,*,#12428,.F.);
#16831=ORIENTED_EDGE('',*,*,#12430,.F.);
#16832=ORIENTED_EDGE('',*,*,#12431,.T.);
#16833=ORIENTED_EDGE('',*,*,#12429,.F.);
#16834=ORIENTED_EDGE('',*,*,#12431,.F.);
#16835=ORIENTED_EDGE('',*,*,#12396,.T.);
#16836=ORIENTED_EDGE('',*,*,#12432,.T.);
#16837=ORIENTED_EDGE('',*,*,#12430,.T.);
#16838=ORIENTED_EDGE('',*,*,#12432,.F.);
#16839=ORIENTED_EDGE('',*,*,#12433,.F.);
#16840=ORIENTED_EDGE('',*,*,#12434,.F.);
#16841=ORIENTED_EDGE('',*,*,#12435,.T.);
#16842=ORIENTED_EDGE('',*,*,#12385,.F.);
#16843=ORIENTED_EDGE('',*,*,#12435,.F.);
#16844=ORIENTED_EDGE('',*,*,#12436,.T.);
#16845=ORIENTED_EDGE('',*,*,#12437,.T.);
#16846=ORIENTED_EDGE('',*,*,#12438,.T.);
#16847=ORIENTED_EDGE('',*,*,#12437,.F.);
#16848=ORIENTED_EDGE('',*,*,#12439,.F.);
#16849=ORIENTED_EDGE('',*,*,#12440,.T.);
#16850=ORIENTED_EDGE('',*,*,#12438,.F.);
#16851=ORIENTED_EDGE('',*,*,#12440,.F.);
#16852=ORIENTED_EDGE('',*,*,#12379,.F.);
#16853=ORIENTED_EDGE('',*,*,#12441,.F.);
#16854=ORIENTED_EDGE('',*,*,#12442,.F.);
#16855=ORIENTED_EDGE('',*,*,#12443,.F.);
#16856=ORIENTED_EDGE('',*,*,#12392,.F.);
#16857=ORIENTED_EDGE('',*,*,#12444,.F.);
#16858=ORIENTED_EDGE('',*,*,#12445,.F.);
#16859=ORIENTED_EDGE('',*,*,#12446,.F.);
#16860=ORIENTED_EDGE('',*,*,#12436,.F.);
#16861=ORIENTED_EDGE('',*,*,#12447,.T.);
#16862=ORIENTED_EDGE('',*,*,#12448,.T.);
#16863=ORIENTED_EDGE('',*,*,#12449,.T.);
#16864=ORIENTED_EDGE('',*,*,#12448,.F.);
#16865=ORIENTED_EDGE('',*,*,#12449,.F.);
#16866=ORIENTED_EDGE('',*,*,#12450,.T.);
#16867=ORIENTED_EDGE('',*,*,#12451,.T.);
#16868=ORIENTED_EDGE('',*,*,#12450,.F.);
#16869=ORIENTED_EDGE('',*,*,#12377,.F.);
#16870=ORIENTED_EDGE('',*,*,#12452,.F.);
#16871=ORIENTED_EDGE('',*,*,#12453,.F.);
#16872=ORIENTED_EDGE('',*,*,#12454,.F.);
#16873=ORIENTED_EDGE('',*,*,#12390,.F.);
#16874=ORIENTED_EDGE('',*,*,#12455,.F.);
#16875=ORIENTED_EDGE('',*,*,#12456,.F.);
#16876=ORIENTED_EDGE('',*,*,#12457,.F.);
#16877=ORIENTED_EDGE('',*,*,#12447,.F.);
#16878=ORIENTED_EDGE('',*,*,#12458,.F.);
#16879=ORIENTED_EDGE('',*,*,#12459,.T.);
#16880=ORIENTED_EDGE('',*,*,#12460,.F.);
#16881=ORIENTED_EDGE('',*,*,#12461,.F.);
#16882=ORIENTED_EDGE('',*,*,#12462,.T.);
#16883=ORIENTED_EDGE('',*,*,#12463,.F.);
#16884=ORIENTED_EDGE('',*,*,#12464,.F.);
#16885=ORIENTED_EDGE('',*,*,#12459,.F.);
#16886=ORIENTED_EDGE('',*,*,#12465,.F.);
#16887=ORIENTED_EDGE('',*,*,#12466,.T.);
#16888=ORIENTED_EDGE('',*,*,#12467,.T.);
#16889=ORIENTED_EDGE('',*,*,#12451,.F.);
#16890=ORIENTED_EDGE('',*,*,#12458,.T.);
#16891=ORIENTED_EDGE('',*,*,#12468,.F.);
#16892=ORIENTED_EDGE('',*,*,#12469,.F.);
#16893=ORIENTED_EDGE('',*,*,#12462,.F.);
#16894=ORIENTED_EDGE('',*,*,#12470,.F.);
#16895=ORIENTED_EDGE('',*,*,#12471,.F.);
#16896=ORIENTED_EDGE('',*,*,#12467,.F.);
#16897=ORIENTED_EDGE('',*,*,#12472,.T.);
#16898=ORIENTED_EDGE('',*,*,#12472,.F.);
#16899=ORIENTED_EDGE('',*,*,#12466,.F.);
#16900=ORIENTED_EDGE('',*,*,#12468,.T.);
#16901=ORIENTED_EDGE('',*,*,#12465,.T.);
#16902=ORIENTED_EDGE('',*,*,#12471,.T.);
#16903=ORIENTED_EDGE('',*,*,#12473,.T.);
#16904=ORIENTED_EDGE('',*,*,#12474,.F.);
#16905=ORIENTED_EDGE('',*,*,#12401,.F.);
#16906=ORIENTED_EDGE('',*,*,#12475,.T.);
#16907=ORIENTED_EDGE('',*,*,#12476,.T.);
#16908=ORIENTED_EDGE('',*,*,#12470,.T.);
#16909=ORIENTED_EDGE('',*,*,#12461,.T.);
#16910=ORIENTED_EDGE('',*,*,#12477,.F.);
#16911=ORIENTED_EDGE('',*,*,#12478,.F.);
#16912=ORIENTED_EDGE('',*,*,#12473,.F.);
#16913=ORIENTED_EDGE('',*,*,#12454,.T.);
#16914=ORIENTED_EDGE('',*,*,#12479,.F.);
#16915=ORIENTED_EDGE('',*,*,#12444,.T.);
#16916=ORIENTED_EDGE('',*,*,#12391,.T.);
#16917=ORIENTED_EDGE('',*,*,#12453,.T.);
#16918=ORIENTED_EDGE('',*,*,#12480,.F.);
#16919=ORIENTED_EDGE('',*,*,#12445,.T.);
#16920=ORIENTED_EDGE('',*,*,#12479,.T.);
#16921=ORIENTED_EDGE('',*,*,#12452,.T.);
#16922=ORIENTED_EDGE('',*,*,#12380,.F.);
#16923=ORIENTED_EDGE('',*,*,#12446,.T.);
#16924=ORIENTED_EDGE('',*,*,#12480,.T.);
#16925=ORIENTED_EDGE('',*,*,#12481,.F.);
#16926=ORIENTED_EDGE('',*,*,#12482,.F.);
#16927=ORIENTED_EDGE('',*,*,#12483,.T.);
#16928=ORIENTED_EDGE('',*,*,#12484,.T.);
#16929=ORIENTED_EDGE('',*,*,#12483,.F.);
#16930=ORIENTED_EDGE('',*,*,#12485,.F.);
#16931=ORIENTED_EDGE('',*,*,#12486,.F.);
#16932=ORIENTED_EDGE('',*,*,#12487,.F.);
#16933=ORIENTED_EDGE('',*,*,#12433,.T.);
#16934=ORIENTED_EDGE('',*,*,#12434,.T.);
#16935=ORIENTED_EDGE('',*,*,#12488,.F.);
#16936=ORIENTED_EDGE('',*,*,#12489,.F.);
#16937=ORIENTED_EDGE('',*,*,#12490,.F.);
#16938=ORIENTED_EDGE('',*,*,#12491,.T.);
#16939=ORIENTED_EDGE('',*,*,#12489,.T.);
#16940=ORIENTED_EDGE('',*,*,#12492,.F.);
#16941=ORIENTED_EDGE('',*,*,#12493,.F.);
#16942=ORIENTED_EDGE('',*,*,#12487,.T.);
#16943=ORIENTED_EDGE('',*,*,#12494,.F.);
#16944=ORIENTED_EDGE('',*,*,#12495,.F.);
#16945=ORIENTED_EDGE('',*,*,#12490,.T.);
#16946=ORIENTED_EDGE('',*,*,#12491,.F.);
#16947=ORIENTED_EDGE('',*,*,#12439,.T.);
#16948=ORIENTED_EDGE('',*,*,#12484,.F.);
#16949=ORIENTED_EDGE('',*,*,#12492,.T.);
#16950=ORIENTED_EDGE('',*,*,#12488,.T.);
#16951=ORIENTED_EDGE('',*,*,#12495,.T.);
#16952=ORIENTED_EDGE('',*,*,#12496,.T.);
#16953=ORIENTED_EDGE('',*,*,#12497,.F.);
#16954=ORIENTED_EDGE('',*,*,#12397,.F.);
#16955=ORIENTED_EDGE('',*,*,#12498,.T.);
#16956=ORIENTED_EDGE('',*,*,#12499,.T.);
#16957=ORIENTED_EDGE('',*,*,#12494,.T.);
#16958=ORIENTED_EDGE('',*,*,#12486,.T.);
#16959=ORIENTED_EDGE('',*,*,#12500,.F.);
#16960=ORIENTED_EDGE('',*,*,#12501,.F.);
#16961=ORIENTED_EDGE('',*,*,#12496,.F.);
#16962=ORIENTED_EDGE('',*,*,#12400,.F.);
#16963=ORIENTED_EDGE('',*,*,#12502,.T.);
#16964=ORIENTED_EDGE('',*,*,#12503,.T.);
#16965=ORIENTED_EDGE('',*,*,#12498,.F.);
#16966=ORIENTED_EDGE('',*,*,#12485,.T.);
#16967=ORIENTED_EDGE('',*,*,#12482,.T.);
#16968=ORIENTED_EDGE('',*,*,#12504,.T.);
#16969=ORIENTED_EDGE('',*,*,#12502,.F.);
#16970=ORIENTED_EDGE('',*,*,#12399,.F.);
#16971=ORIENTED_EDGE('',*,*,#12505,.T.);
#16972=ORIENTED_EDGE('',*,*,#12500,.T.);
#16973=ORIENTED_EDGE('',*,*,#12398,.F.);
#16974=ORIENTED_EDGE('',*,*,#12497,.T.);
#16975=ORIENTED_EDGE('',*,*,#12501,.T.);
#16976=ORIENTED_EDGE('',*,*,#12505,.F.);
#16977=ORIENTED_EDGE('',*,*,#12493,.T.);
#16978=ORIENTED_EDGE('',*,*,#12499,.F.);
#16979=ORIENTED_EDGE('',*,*,#12503,.F.);
#16980=ORIENTED_EDGE('',*,*,#12504,.F.);
#16981=ORIENTED_EDGE('',*,*,#12481,.T.);
#16982=ORIENTED_EDGE('',*,*,#12404,.F.);
#16983=ORIENTED_EDGE('',*,*,#12506,.T.);
#16984=ORIENTED_EDGE('',*,*,#12507,.T.);
#16985=ORIENTED_EDGE('',*,*,#12475,.F.);
#16986=ORIENTED_EDGE('',*,*,#12460,.T.);
#16987=ORIENTED_EDGE('',*,*,#12464,.T.);
#16988=ORIENTED_EDGE('',*,*,#12508,.T.);
#16989=ORIENTED_EDGE('',*,*,#12506,.F.);
#16990=ORIENTED_EDGE('',*,*,#12403,.F.);
#16991=ORIENTED_EDGE('',*,*,#12509,.T.);
#16992=ORIENTED_EDGE('',*,*,#12477,.T.);
#16993=ORIENTED_EDGE('',*,*,#12402,.F.);
#16994=ORIENTED_EDGE('',*,*,#12474,.T.);
#16995=ORIENTED_EDGE('',*,*,#12478,.T.);
#16996=ORIENTED_EDGE('',*,*,#12509,.F.);
#16997=ORIENTED_EDGE('',*,*,#12469,.T.);
#16998=ORIENTED_EDGE('',*,*,#12476,.F.);
#16999=ORIENTED_EDGE('',*,*,#12507,.F.);
#17000=ORIENTED_EDGE('',*,*,#12508,.F.);
#17001=ORIENTED_EDGE('',*,*,#12463,.T.);
#17002=ORIENTED_EDGE('',*,*,#12405,.T.);
#17003=ORIENTED_EDGE('',*,*,#12510,.T.);
#17004=ORIENTED_EDGE('',*,*,#12511,.T.);
#17005=ORIENTED_EDGE('',*,*,#12512,.T.);
#17006=ORIENTED_EDGE('',*,*,#12510,.F.);
#17007=ORIENTED_EDGE('',*,*,#12513,.F.);
#17008=ORIENTED_EDGE('',*,*,#12514,.F.);
#17009=ORIENTED_EDGE('',*,*,#12515,.T.);
#17010=ORIENTED_EDGE('',*,*,#12511,.F.);
#17011=ORIENTED_EDGE('',*,*,#12512,.F.);
#17012=ORIENTED_EDGE('',*,*,#12515,.F.);
#17013=ORIENTED_EDGE('',*,*,#12513,.T.);
#17014=ORIENTED_EDGE('',*,*,#12514,.T.);
#17015=ORIENTED_EDGE('',*,*,#12516,.T.);
#17016=ORIENTED_EDGE('',*,*,#12384,.T.);
#17017=ORIENTED_EDGE('',*,*,#12516,.F.);
#17018=ORIENTED_EDGE('',*,*,#12455,.T.);
#17019=ORIENTED_EDGE('',*,*,#12393,.T.);
#17020=ORIENTED_EDGE('',*,*,#12443,.T.);
#17021=ORIENTED_EDGE('',*,*,#12517,.F.);
#17022=ORIENTED_EDGE('',*,*,#12456,.T.);
#17023=ORIENTED_EDGE('',*,*,#12517,.T.);
#17024=ORIENTED_EDGE('',*,*,#12442,.T.);
#17025=ORIENTED_EDGE('',*,*,#12518,.F.);
#17026=ORIENTED_EDGE('',*,*,#12457,.T.);
#17027=ORIENTED_EDGE('',*,*,#12518,.T.);
#17028=ORIENTED_EDGE('',*,*,#12441,.T.);
#17029=ORIENTED_EDGE('',*,*,#12378,.F.);
#21381=CONICAL_SURFACE('',#23867,0.465,0.785398163397456);
#21382=CONICAL_SURFACE('',#23882,0.465,0.785398163397452);
#21383=CONICAL_SURFACE('',#23901,0.465,0.785398163397448);
#21384=CONICAL_SURFACE('',#23905,0.465,0.785398163397444);
#21385=CONICAL_SURFACE('',#23906,0.465,0.785398163397448);
#21386=CONICAL_SURFACE('',#23910,0.465,0.785398163397444);
#21387=CONICAL_SURFACE('',#23911,0.465,0.785398163397456);
#21388=CONICAL_SURFACE('',#23915,0.465,0.785398163397452);
#21389=CONICAL_SURFACE('',#23916,0.465,0.785398163397448);
#21390=CONICAL_SURFACE('',#23920,0.465,0.785398163397444);
#21391=CONICAL_SURFACE('',#23921,0.465,0.785398163397448);
#21392=CONICAL_SURFACE('',#23925,0.465,0.785398163397444);
#21393=CONICAL_SURFACE('',#23927,0.8781,0.785398163397448);
#21394=CONICAL_SURFACE('',#23933,0.8781,0.785398163397448);
#21395=CONICAL_SURFACE('',#23946,0.6,1.02974425867665);
#21396=CONICAL_SURFACE('',#23953,6.95,0.785398163397447);
#21397=CONICAL_SURFACE('',#23957,6.95,0.785398163397446);
#21398=CONICAL_SURFACE('',#23964,0.3,1.02974425867665);
#21399=CONICAL_SURFACE('',#23984,1.525,0.785398163397448);
#21400=CONICAL_SURFACE('',#23990,1.525,0.785398163397451);
#21401=CONICAL_SURFACE('',#23991,6.95,0.785398163397447);
#21402=CONICAL_SURFACE('',#23995,6.95,0.785398163397446);
#21937=ADVANCED_FACE('',(#3107),#21381,.F.);
#21938=ADVANCED_FACE('',(#3108),#2529,.F.);
#21939=ADVANCED_FACE('',(#3109,#1694,#1695,#1696,#1697,#1698,#1699,#1700,
#1701),#2041,.T.);
#21940=ADVANCED_FACE('',(#3110),#21382,.F.);
#21941=ADVANCED_FACE('',(#3111,#1702,#1703,#1704,#1705,#1706,#1707,#1708,
#1709,#1710),#2042,.T.);
#21942=ADVANCED_FACE('',(#3112),#21383,.F.);
#21943=ADVANCED_FACE('',(#3113),#2530,.F.);
#21944=ADVANCED_FACE('',(#3114),#21384,.F.);
#21945=ADVANCED_FACE('',(#3115),#21385,.F.);
#21946=ADVANCED_FACE('',(#3116),#2531,.F.);
#21947=ADVANCED_FACE('',(#3117),#21386,.F.);
#21948=ADVANCED_FACE('',(#3118),#21387,.F.);
#21949=ADVANCED_FACE('',(#3119),#2532,.F.);
#21950=ADVANCED_FACE('',(#3120),#21388,.F.);
#21951=ADVANCED_FACE('',(#3121),#21389,.F.);
#21952=ADVANCED_FACE('',(#3122),#2533,.F.);
#21953=ADVANCED_FACE('',(#3123),#21390,.F.);
#21954=ADVANCED_FACE('',(#3124),#21391,.F.);
#21955=ADVANCED_FACE('',(#3125),#2534,.F.);
#21956=ADVANCED_FACE('',(#3126),#21392,.F.);
#21957=ADVANCED_FACE('',(#3127),#2535,.F.);
#21958=ADVANCED_FACE('',(#3128),#21393,.F.);
#21959=ADVANCED_FACE('',(#3129),#2536,.F.);
#21960=ADVANCED_FACE('',(#3130,#1711),#2043,.T.);
#21961=ADVANCED_FACE('',(#3131),#21394,.F.);
#21962=ADVANCED_FACE('',(#3132),#2537,.F.);
#21963=ADVANCED_FACE('',(#3133,#1712),#2044,.F.);
#21964=ADVANCED_FACE('',(#3134),#2538,.F.);
#21965=ADVANCED_FACE('',(#3135),#2539,.F.);
#21966=ADVANCED_FACE('',(#3136,#1713),#2045,.F.);
#21967=ADVANCED_FACE('',(#3137),#21395,.F.);
#21968=ADVANCED_FACE('',(#3138),#2540,.T.);
#21969=ADVANCED_FACE('',(#3139),#2046,.F.);
#21970=ADVANCED_FACE('',(#3140),#21396,.T.);
#21971=ADVANCED_FACE('',(#3141),#2541,.T.);
#21972=ADVANCED_FACE('',(#3142),#21397,.T.);
#21973=ADVANCED_FACE('',(#3143,#1714),#2542,.F.);
#21974=ADVANCED_FACE('',(#3144),#2543,.F.);
#21975=ADVANCED_FACE('',(#3145),#21398,.F.);
#21976=ADVANCED_FACE('',(#3146,#1715),#2047,.F.);
#21977=ADVANCED_FACE('',(#3147),#2544,.T.);
#21978=ADVANCED_FACE('',(#3148),#2048,.F.);
#21979=ADVANCED_FACE('',(#3149),#2545,.F.);
#21980=ADVANCED_FACE('',(#3150),#2546,.F.);
#21981=ADVANCED_FACE('',(#3151),#2547,.F.);
#21982=ADVANCED_FACE('',(#3152),#2049,.F.);
#21983=ADVANCED_FACE('',(#3153),#2548,.F.);
#21984=ADVANCED_FACE('',(#3154),#2549,.F.);
#21985=ADVANCED_FACE('',(#3155),#2550,.F.);
#21986=ADVANCED_FACE('',(#3156),#2050,.F.);
#21987=ADVANCED_FACE('',(#3157),#21399,.F.);
#21988=ADVANCED_FACE('',(#3158),#2551,.F.);
#21989=ADVANCED_FACE('',(#3159),#21400,.F.);
#21990=ADVANCED_FACE('',(#3160),#21401,.T.);
#21991=ADVANCED_FACE('',(#3161),#2552,.T.);
#21992=ADVANCED_FACE('',(#3162),#21402,.T.);
#22815=CLOSED_SHELL('',(#21937,#21938,#21939,#21940,#21941,#21942,#21943,
#21944,#21945,#21946,#21947,#21948,#21949,#21950,#21951,#21952,#21953,#21954,
#21955,#21956,#21957,#21958,#21959,#21960,#21961,#21962,#21963,#21964,#21965,
#21966,#21967,#21968,#21969,#21970,#21971,#21972,#21973,#21974,#21975,#21976,
#21977,#21978,#21979,#21980,#21981,#21982,#21983,#21984,#21985,#21986,#21987,
#21988,#21989,#21990,#21991,#21992));
#23866=AXIS2_PLACEMENT_3D('',#42776,#27241,#27242);
#23867=AXIS2_PLACEMENT_3D('',#42777,#27243,#27244);
#23868=AXIS2_PLACEMENT_3D('',#42779,#27245,#27246);
#23869=AXIS2_PLACEMENT_3D('',#42782,#27248,#27249);
#23870=AXIS2_PLACEMENT_3D('',#42783,#27250,#27251);
#23871=AXIS2_PLACEMENT_3D('',#42785,#27252,#27253);
#23872=AXIS2_PLACEMENT_3D('',#42787,#27255,#27256);
#23873=AXIS2_PLACEMENT_3D('',#42792,#27258,#27259);
#23874=AXIS2_PLACEMENT_3D('',#42795,#27261,#27262);
#23875=AXIS2_PLACEMENT_3D('',#42797,#27263,#27264);
#23876=AXIS2_PLACEMENT_3D('',#42799,#27265,#27266);
#23877=AXIS2_PLACEMENT_3D('',#42801,#27267,#27268);
#23878=AXIS2_PLACEMENT_3D('',#42803,#27269,#27270);
#23879=AXIS2_PLACEMENT_3D('',#42805,#27271,#27272);
#23880=AXIS2_PLACEMENT_3D('',#42807,#27273,#27274);
#23881=AXIS2_PLACEMENT_3D('',#42809,#27275,#27276);
#23882=AXIS2_PLACEMENT_3D('',#42810,#27277,#27278);
#23883=AXIS2_PLACEMENT_3D('',#42812,#27279,#27280);
#23884=AXIS2_PLACEMENT_3D('',#42814,#27282,#27283);
#23885=AXIS2_PLACEMENT_3D('',#42819,#27285,#27286);
#23886=AXIS2_PLACEMENT_3D('',#42822,#27288,#27289);
#23887=AXIS2_PLACEMENT_3D('',#42824,#27290,#27291);
#23888=AXIS2_PLACEMENT_3D('',#42826,#27292,#27293);
#23889=AXIS2_PLACEMENT_3D('',#42828,#27294,#27295);
#23890=AXIS2_PLACEMENT_3D('',#42831,#27296,#27297);
#23891=AXIS2_PLACEMENT_3D('',#42833,#27298,#27299);
#23892=AXIS2_PLACEMENT_3D('',#42835,#27300,#27301);
#23893=AXIS2_PLACEMENT_3D('',#42836,#27302,#27303);
#23894=AXIS2_PLACEMENT_3D('',#42839,#27304,#27305);
#23895=AXIS2_PLACEMENT_3D('',#42841,#27306,#27307);
#23896=AXIS2_PLACEMENT_3D('',#42843,#27308,#27309);
#23897=AXIS2_PLACEMENT_3D('',#42844,#27310,#27311);
#23898=AXIS2_PLACEMENT_3D('',#42846,#27312,#27313);
#23899=AXIS2_PLACEMENT_3D('',#42848,#27314,#27315);
#23900=AXIS2_PLACEMENT_3D('',#42850,#27316,#27317);
#23901=AXIS2_PLACEMENT_3D('',#42851,#27318,#27319);
#23902=AXIS2_PLACEMENT_3D('',#42854,#27321,#27322);
#23903=AXIS2_PLACEMENT_3D('',#42855,#27323,#27324);
#23904=AXIS2_PLACEMENT_3D('',#42857,#27325,#27326);
#23905=AXIS2_PLACEMENT_3D('',#42859,#27328,#27329);
#23906=AXIS2_PLACEMENT_3D('',#42861,#27331,#27332);
#23907=AXIS2_PLACEMENT_3D('',#42864,#27334,#27335);
#23908=AXIS2_PLACEMENT_3D('',#42865,#27336,#27337);
#23909=AXIS2_PLACEMENT_3D('',#42867,#27338,#27339);
#23910=AXIS2_PLACEMENT_3D('',#42869,#27341,#27342);
#23911=AXIS2_PLACEMENT_3D('',#42871,#27344,#27345);
#23912=AXIS2_PLACEMENT_3D('',#42874,#27347,#27348);
#23913=AXIS2_PLACEMENT_3D('',#42875,#27349,#27350);
#23914=AXIS2_PLACEMENT_3D('',#42877,#27351,#27352);
#23915=AXIS2_PLACEMENT_3D('',#42879,#27354,#27355);
#23916=AXIS2_PLACEMENT_3D('',#42881,#27357,#27358);
#23917=AXIS2_PLACEMENT_3D('',#42884,#27360,#27361);
#23918=AXIS2_PLACEMENT_3D('',#42885,#27362,#27363);
#23919=AXIS2_PLACEMENT_3D('',#42887,#27364,#27365);
#23920=AXIS2_PLACEMENT_3D('',#42889,#27367,#27368);
#23921=AXIS2_PLACEMENT_3D('',#42891,#27370,#27371);
#23922=AXIS2_PLACEMENT_3D('',#42894,#27373,#27374);
#23923=AXIS2_PLACEMENT_3D('',#42895,#27375,#27376);
#23924=AXIS2_PLACEMENT_3D('',#42897,#27377,#27378);
#23925=AXIS2_PLACEMENT_3D('',#42899,#27380,#27381);
#23926=AXIS2_PLACEMENT_3D('',#42901,#27383,#27384);
#23927=AXIS2_PLACEMENT_3D('',#42941,#27386,#27387);
#23928=AXIS2_PLACEMENT_3D('',#42943,#27388,#27389);
#23929=AXIS2_PLACEMENT_3D('',#42946,#27391,#27392);
#23930=AXIS2_PLACEMENT_3D('',#42947,#27393,#27394);
#23931=AXIS2_PLACEMENT_3D('',#42949,#27395,#27396);
#23932=AXIS2_PLACEMENT_3D('',#42951,#27398,#27399);
#23933=AXIS2_PLACEMENT_3D('',#42970,#27402,#27403);
#23934=AXIS2_PLACEMENT_3D('',#42972,#27404,#27405);
#23935=AXIS2_PLACEMENT_3D('',#42975,#27407,#27408);
#23936=AXIS2_PLACEMENT_3D('',#42976,#27409,#27410);
#23937=AXIS2_PLACEMENT_3D('',#42979,#27412,#27413);
#23938=AXIS2_PLACEMENT_3D('',#42980,#27414,#27415);
#23939=AXIS2_PLACEMENT_3D('',#42999,#27418,#27419);
#23940=AXIS2_PLACEMENT_3D('',#43001,#27420,#27421);
#23941=AXIS2_PLACEMENT_3D('',#43018,#27424,#27425);
#23942=AXIS2_PLACEMENT_3D('',#43031,#27427,#27428);
#23943=AXIS2_PLACEMENT_3D('',#43049,#27429,#27430);
#23944=AXIS2_PLACEMENT_3D('',#43050,#27431,#27432);
#23945=AXIS2_PLACEMENT_3D('',#43051,#27433,#27434);
#23946=AXIS2_PLACEMENT_3D('',#43052,#27435,#27436);
#23947=AXIS2_PLACEMENT_3D('',#43075,#27438,#27439);
#23948=AXIS2_PLACEMENT_3D('',#43077,#27440,#27441);
#23949=AXIS2_PLACEMENT_3D('',#43081,#27444,#27445);
#23950=AXIS2_PLACEMENT_3D('',#43082,#27446,#27447);
#23951=AXIS2_PLACEMENT_3D('',#43084,#27448,#27449);
#23952=AXIS2_PLACEMENT_3D('',#43085,#27450,#27451);
#23953=AXIS2_PLACEMENT_3D('',#43086,#27452,#27453);
#23954=AXIS2_PLACEMENT_3D('',#43087,#27454,#27455);
#23955=AXIS2_PLACEMENT_3D('',#43088,#27456,#27457);
#23956=AXIS2_PLACEMENT_3D('',#43089,#27458,#27459);
#23957=AXIS2_PLACEMENT_3D('',#43090,#27460,#27461);
#23958=AXIS2_PLACEMENT_3D('',#43091,#27462,#27463);
#23959=AXIS2_PLACEMENT_3D('',#43108,#27466,#27467);
#23960=AXIS2_PLACEMENT_3D('',#43122,#27469,#27470);
#23961=AXIS2_PLACEMENT_3D('',#43123,#27471,#27472);
#23962=AXIS2_PLACEMENT_3D('',#43141,#27473,#27474);
#23963=AXIS2_PLACEMENT_3D('',#43142,#27475,#27476);
#23964=AXIS2_PLACEMENT_3D('',#43143,#27477,#27478);
#23965=AXIS2_PLACEMENT_3D('',#43166,#27480,#27481);
#23966=AXIS2_PLACEMENT_3D('',#43167,#27482,#27483);
#23967=AXIS2_PLACEMENT_3D('',#43169,#27484,#27485);
#23968=AXIS2_PLACEMENT_3D('',#43173,#27488,#27489);
#23969=AXIS2_PLACEMENT_3D('',#43174,#27490,#27491);
#23970=AXIS2_PLACEMENT_3D('',#43176,#27492,#27493);
#23971=AXIS2_PLACEMENT_3D('',#43177,#27494,#27495);
#23972=AXIS2_PLACEMENT_3D('',#43178,#27496,#27497);
#23973=AXIS2_PLACEMENT_3D('',#43181,#27499,#27500);
#23974=AXIS2_PLACEMENT_3D('',#43182,#27501,#27502);
#23975=AXIS2_PLACEMENT_3D('',#43183,#27503,#27504);
#23976=AXIS2_PLACEMENT_3D('',#43185,#27506,#27507);
#23977=AXIS2_PLACEMENT_3D('',#43186,#27508,#27509);
#23978=AXIS2_PLACEMENT_3D('',#43187,#27510,#27511);
#23979=AXIS2_PLACEMENT_3D('',#43190,#27513,#27514);
#23980=AXIS2_PLACEMENT_3D('',#43191,#27515,#27516);
#23981=AXIS2_PLACEMENT_3D('',#43192,#27517,#27518);
#23982=AXIS2_PLACEMENT_3D('',#43194,#27520,#27521);
#23983=AXIS2_PLACEMENT_3D('',#43195,#27522,#27523);
#23984=AXIS2_PLACEMENT_3D('',#43196,#27524,#27525);
#23985=AXIS2_PLACEMENT_3D('',#43200,#27527,#27528);
#23986=AXIS2_PLACEMENT_3D('',#43201,#27529,#27530);
#23987=AXIS2_PLACEMENT_3D('',#43202,#27531,#27532);
#23988=AXIS2_PLACEMENT_3D('',#43205,#27533,#27534);
#23989=AXIS2_PLACEMENT_3D('',#43206,#27535,#27536);
#23990=AXIS2_PLACEMENT_3D('',#43208,#27538,#27539);
#23991=AXIS2_PLACEMENT_3D('',#43210,#27541,#27542);
#23992=AXIS2_PLACEMENT_3D('',#43211,#27543,#27544);
#23993=AXIS2_PLACEMENT_3D('',#43212,#27545,#27546);
#23994=AXIS2_PLACEMENT_3D('',#43213,#27547,#27548);
#23995=AXIS2_PLACEMENT_3D('',#43214,#27549,#27550);
#27241=DIRECTION('axis',(0.,0.,1.));
#27242=DIRECTION('refdir',(1.,0.,0.));
#27243=DIRECTION('center_axis',(0.,0.,1.));
#27244=DIRECTION('ref_axis',(1.,0.,0.));
#27245=DIRECTION('center_axis',(0.,0.,1.));
#27246=DIRECTION('ref_axis',(1.,0.,0.));
#27247=DIRECTION('',(0.707106781186553,8.659560562355E-17,-0.707106781186542));
#27248=DIRECTION('center_axis',(0.,0.,-1.));
#27249=DIRECTION('ref_axis',(1.,0.,0.));
#27250=DIRECTION('center_axis',(0.,0.,1.));
#27251=DIRECTION('ref_axis',(1.,0.,0.));
#27252=DIRECTION('center_axis',(0.,0.,1.));
#27253=DIRECTION('ref_axis',(1.,0.,0.));
#27254=DIRECTION('',(0.,0.,1.));
#27255=DIRECTION('center_axis',(0.,0.,1.));
#27256=DIRECTION('ref_axis',(1.,0.,0.));
#27257=DIRECTION('',(1.,0.,0.));
#27258=DIRECTION('center_axis',(0.,0.,1.));
#27259=DIRECTION('ref_axis',(1.,0.,0.));
#27260=DIRECTION('',(-1.,0.,0.));
#27261=DIRECTION('center_axis',(0.,0.,1.));
#27262=DIRECTION('ref_axis',(1.,0.,0.));
#27263=DIRECTION('center_axis',(0.,0.,1.));
#27264=DIRECTION('ref_axis',(1.,0.,0.));
#27265=DIRECTION('center_axis',(0.,0.,1.));
#27266=DIRECTION('ref_axis',(1.,0.,0.));
#27267=DIRECTION('center_axis',(0.,0.,1.));
#27268=DIRECTION('ref_axis',(1.,0.,0.));
#27269=DIRECTION('center_axis',(0.,0.,1.));
#27270=DIRECTION('ref_axis',(-1.,0.,0.));
#27271=DIRECTION('center_axis',(0.,0.,-1.));
#27272=DIRECTION('ref_axis',(1.,0.,0.));
#27273=DIRECTION('center_axis',(0.,0.,1.));
#27274=DIRECTION('ref_axis',(1.,0.,0.));
#27275=DIRECTION('center_axis',(0.,0.,1.));
#27276=DIRECTION('ref_axis',(1.,0.,0.));
#27277=DIRECTION('center_axis',(0.,0.,-1.));
#27278=DIRECTION('ref_axis',(1.,0.,0.));
#27279=DIRECTION('center_axis',(0.,0.,-1.));
#27280=DIRECTION('ref_axis',(1.,0.,0.));
#27281=DIRECTION('',(0.70710678118655,-8.65956056235496E-17,0.707106781186545));
#27282=DIRECTION('center_axis',(0.,0.,-1.));
#27283=DIRECTION('ref_axis',(-1.,0.,0.));
#27284=DIRECTION('',(-1.,0.,0.));
#27285=DIRECTION('center_axis',(0.,0.,1.));
#27286=DIRECTION('ref_axis',(1.,0.,0.));
#27287=DIRECTION('',(1.,0.,0.));
#27288=DIRECTION('center_axis',(0.,0.,1.));
#27289=DIRECTION('ref_axis',(1.,0.,0.));
#27290=DIRECTION('center_axis',(0.,0.,-1.));
#27291=DIRECTION('ref_axis',(1.,0.,0.));
#27292=DIRECTION('center_axis',(0.,0.,-1.));
#27293=DIRECTION('ref_axis',(1.,0.,0.));
#27294=DIRECTION('center_axis',(0.,0.,-1.));
#27295=DIRECTION('ref_axis',(1.,0.,0.));
#27296=DIRECTION('center_axis',(0.,0.,-1.));
#27297=DIRECTION('ref_axis',(0.819152044288992,0.573576436351046,0.));
#27298=DIRECTION('center_axis',(0.,0.,1.));
#27299=DIRECTION('ref_axis',(-0.819152044288992,-0.573576436351046,0.));
#27300=DIRECTION('center_axis',(0.,0.,1.));
#27301=DIRECTION('ref_axis',(0.819152044288992,0.573576436351046,0.));
#27302=DIRECTION('center_axis',(0.,0.,1.));
#27303=DIRECTION('ref_axis',(-0.819152044288991,0.573576436351046,0.));
#27304=DIRECTION('center_axis',(0.,0.,-1.));
#27305=DIRECTION('ref_axis',(-0.819152044288992,-0.573576436351046,0.));
#27306=DIRECTION('center_axis',(0.,0.,1.));
#27307=DIRECTION('ref_axis',(0.819152044288991,0.573576436351047,0.));
#27308=DIRECTION('center_axis',(0.,0.,1.));
#27309=DIRECTION('ref_axis',(-0.819152044288992,-0.573576436351046,0.));
#27310=DIRECTION('center_axis',(0.,0.,1.));
#27311=DIRECTION('ref_axis',(0.819152044288992,-0.573576436351046,0.));
#27312=DIRECTION('center_axis',(0.,0.,-1.));
#27313=DIRECTION('ref_axis',(-1.,0.,0.));
#27314=DIRECTION('center_axis',(0.,0.,-1.));
#27315=DIRECTION('ref_axis',(1.,0.,0.));
#27316=DIRECTION('center_axis',(0.,0.,-1.));
#27317=DIRECTION('ref_axis',(1.,0.,0.));
#27318=DIRECTION('center_axis',(0.,0.,1.));
#27319=DIRECTION('ref_axis',(1.,0.,0.));
#27320=DIRECTION('',(0.707106781186547,8.65956056235493E-17,-0.707106781186547));
#27321=DIRECTION('center_axis',(0.,0.,-1.));
#27322=DIRECTION('ref_axis',(1.,0.,0.));
#27323=DIRECTION('center_axis',(0.,0.,1.));
#27324=DIRECTION('ref_axis',(1.,0.,0.));
#27325=DIRECTION('center_axis',(0.,0.,1.));
#27326=DIRECTION('ref_axis',(1.,0.,0.));
#27327=DIRECTION('',(0.,0.,1.));
#27328=DIRECTION('center_axis',(0.,0.,-1.));
#27329=DIRECTION('ref_axis',(1.,0.,0.));
#27330=DIRECTION('',(0.707106781186545,-8.6595605623549E-17,0.70710678118655));
#27331=DIRECTION('center_axis',(0.,0.,1.));
#27332=DIRECTION('ref_axis',(1.,0.,0.));
#27333=DIRECTION('',(0.707106781186548,8.65956056235493E-17,-0.707106781186548));
#27334=DIRECTION('center_axis',(0.,0.,-1.));
#27335=DIRECTION('ref_axis',(1.,0.,0.));
#27336=DIRECTION('center_axis',(0.,0.,1.));
#27337=DIRECTION('ref_axis',(1.,0.,0.));
#27338=DIRECTION('center_axis',(0.,0.,1.));
#27339=DIRECTION('ref_axis',(1.,0.,0.));
#27340=DIRECTION('',(0.,0.,1.));
#27341=DIRECTION('center_axis',(0.,0.,-1.));
#27342=DIRECTION('ref_axis',(1.,0.,0.));
#27343=DIRECTION('',(0.707106781186545,-8.6595605623549E-17,0.70710678118655));
#27344=DIRECTION('center_axis',(0.,0.,1.));
#27345=DIRECTION('ref_axis',(1.,0.,0.));
#27346=DIRECTION('',(0.707106781186553,8.659560562355E-17,-0.707106781186542));
#27347=DIRECTION('center_axis',(0.,0.,-1.));
#27348=DIRECTION('ref_axis',(1.,0.,0.));
#27349=DIRECTION('center_axis',(0.,0.,1.));
#27350=DIRECTION('ref_axis',(1.,0.,0.));
#27351=DIRECTION('center_axis',(0.,0.,1.));
#27352=DIRECTION('ref_axis',(1.,0.,0.));
#27353=DIRECTION('',(0.,0.,1.));
#27354=DIRECTION('center_axis',(0.,0.,-1.));
#27355=DIRECTION('ref_axis',(1.,0.,0.));
#27356=DIRECTION('',(0.70710678118655,-8.65956056235496E-17,0.707106781186545));
#27357=DIRECTION('center_axis',(0.,0.,1.));
#27358=DIRECTION('ref_axis',(1.,0.,0.));
#27359=DIRECTION('',(0.707106781186547,8.65956056235493E-17,-0.707106781186547));
#27360=DIRECTION('center_axis',(0.,0.,-1.));
#27361=DIRECTION('ref_axis',(1.,0.,0.));
#27362=DIRECTION('center_axis',(0.,0.,1.));
#27363=DIRECTION('ref_axis',(1.,0.,0.));
#27364=DIRECTION('center_axis',(0.,0.,1.));
#27365=DIRECTION('ref_axis',(1.,0.,0.));
#27366=DIRECTION('',(0.,0.,1.));
#27367=DIRECTION('center_axis',(0.,0.,-1.));
#27368=DIRECTION('ref_axis',(1.,0.,0.));
#27369=DIRECTION('',(0.707106781186545,-8.6595605623549E-17,0.70710678118655));
#27370=DIRECTION('center_axis',(0.,0.,1.));
#27371=DIRECTION('ref_axis',(1.,0.,0.));
#27372=DIRECTION('',(0.707106781186547,8.65956056235493E-17,-0.707106781186547));
#27373=DIRECTION('center_axis',(0.,0.,-1.));
#27374=DIRECTION('ref_axis',(1.,0.,0.));
#27375=DIRECTION('center_axis',(0.,0.,1.));
#27376=DIRECTION('ref_axis',(1.,0.,0.));
#27377=DIRECTION('center_axis',(0.,0.,1.));
#27378=DIRECTION('ref_axis',(1.,0.,0.));
#27379=DIRECTION('',(0.,0.,1.));
#27380=DIRECTION('center_axis',(0.,0.,-1.));
#27381=DIRECTION('ref_axis',(1.,0.,0.));
#27382=DIRECTION('',(0.707106781186545,-8.6595605623549E-17,0.70710678118655));
#27383=DIRECTION('center_axis',(0.,0.,1.));
#27384=DIRECTION('ref_axis',(1.,0.,0.));
#27385=DIRECTION('',(0.,0.,1.));
#27386=DIRECTION('center_axis',(0.,1.,0.));
#27387=DIRECTION('ref_axis',(0.,0.,1.));
#27388=DIRECTION('center_axis',(0.,1.,0.));
#27389=DIRECTION('ref_axis',(0.,0.,1.));
#27390=DIRECTION('',(8.65956056235493E-17,-0.707106781186547,0.707106781186547));
#27391=DIRECTION('center_axis',(0.,-1.,0.));
#27392=DIRECTION('ref_axis',(0.,0.,1.));
#27393=DIRECTION('center_axis',(0.,1.,0.));
#27394=DIRECTION('ref_axis',(0.,0.,1.));
#27395=DIRECTION('center_axis',(0.,1.,0.));
#27396=DIRECTION('ref_axis',(1.,0.,0.));
#27397=DIRECTION('',(0.,1.,0.));
#27398=DIRECTION('center_axis',(0.,1.,0.));
#27399=DIRECTION('ref_axis',(1.,0.,0.));
#27400=DIRECTION('',(0.,0.,1.));
#27401=DIRECTION('',(0.,0.,-1.));
#27402=DIRECTION('center_axis',(0.,-1.,0.));
#27403=DIRECTION('ref_axis',(0.,0.,1.));
#27404=DIRECTION('center_axis',(0.,-1.,0.));
#27405=DIRECTION('ref_axis',(0.,0.,1.));
#27406=DIRECTION('',(-8.65956056235493E-17,0.707106781186547,0.707106781186547));
#27407=DIRECTION('center_axis',(0.,1.,0.));
#27408=DIRECTION('ref_axis',(0.,0.,1.));
#27409=DIRECTION('center_axis',(0.,1.,0.));
#27410=DIRECTION('ref_axis',(0.,0.,1.));
#27411=DIRECTION('',(0.,1.,0.));
#27412=DIRECTION('center_axis',(0.,1.,0.));
#27413=DIRECTION('ref_axis',(1.,0.,0.));
#27414=DIRECTION('center_axis',(0.,1.,0.));
#27415=DIRECTION('ref_axis',(1.,0.,0.));
#27416=DIRECTION('',(0.,0.,1.));
#27417=DIRECTION('',(0.,0.,-1.));
#27418=DIRECTION('center_axis',(0.,1.,0.));
#27419=DIRECTION('ref_axis',(0.,0.,1.));
#27420=DIRECTION('center_axis',(0.,1.,0.));
#27421=DIRECTION('ref_axis',(1.,0.,0.));
#27422=DIRECTION('',(0.,1.,0.));
#27423=DIRECTION('',(0.,-1.,0.));
#27424=DIRECTION('center_axis',(0.,1.,0.));
#27425=DIRECTION('ref_axis',(1.,0.,0.));
#27426=DIRECTION('',(0.,1.,0.));
#27427=DIRECTION('center_axis',(0.,1.,0.));
#27428=DIRECTION('ref_axis',(-1.22464679914735E-16,0.,-1.));
#27429=DIRECTION('center_axis',(0.,1.,0.));
#27430=DIRECTION('ref_axis',(1.,0.,0.));
#27431=DIRECTION('center_axis',(0.,1.,0.));
#27432=DIRECTION('ref_axis',(1.,0.,0.));
#27433=DIRECTION('center_axis',(0.,1.,0.));
#27434=DIRECTION('ref_axis',(0.,0.,1.));
#27435=DIRECTION('center_axis',(0.,-1.,0.));
#27436=DIRECTION('ref_axis',(0.,0.,1.));
#27437=DIRECTION('',(1.04972719113862E-16,0.515038074910055,0.857167300702112));
#27438=DIRECTION('center_axis',(0.,0.,1.));
#27439=DIRECTION('ref_axis',(-0.819152044288992,-0.573576436351046,0.));
#27440=DIRECTION('center_axis',(0.,0.,-1.));
#27441=DIRECTION('ref_axis',(-0.819152044288992,-0.573576436351046,0.));
#27442=DIRECTION('',(0.,0.,1.));
#27443=DIRECTION('',(0.,0.,1.));
#27444=DIRECTION('center_axis',(0.,0.,-1.));
#27445=DIRECTION('ref_axis',(-0.819152044288992,-0.573576436351046,0.));
#27446=DIRECTION('center_axis',(0.,0.,1.));
#27447=DIRECTION('ref_axis',(1.,0.,0.));
#27448=DIRECTION('center_axis',(0.,0.,1.));
#27449=DIRECTION('ref_axis',(-0.819152044288992,-0.573576436351046,0.));
#27450=DIRECTION('center_axis',(0.,0.,1.));
#27451=DIRECTION('ref_axis',(0.819152044288991,0.573576436351047,0.));
#27452=DIRECTION('center_axis',(0.,0.,1.));
#27453=DIRECTION('ref_axis',(-1.,-1.22464679914735E-16,0.));
#27454=DIRECTION('center_axis',(0.,0.,1.));
#27455=DIRECTION('ref_axis',(1.,0.,0.));
#27456=DIRECTION('center_axis',(0.,0.,1.));
#27457=DIRECTION('ref_axis',(-1.,-1.22464679914735E-16,0.));
#27458=DIRECTION('center_axis',(0.,0.,1.));
#27459=DIRECTION('ref_axis',(1.,0.,0.));
#27460=DIRECTION('center_axis',(0.,0.,-1.));
#27461=DIRECTION('ref_axis',(-1.,-1.22464679914735E-16,0.));
#27462=DIRECTION('center_axis',(0.,1.,0.));
#27463=DIRECTION('ref_axis',(0.,0.,1.));
#27464=DIRECTION('',(0.,-1.,0.));
#27465=DIRECTION('',(0.,1.,0.));
#27466=DIRECTION('center_axis',(0.,1.,0.));
#27467=DIRECTION('ref_axis',(1.,0.,0.));
#27468=DIRECTION('',(0.,1.,0.));
#27469=DIRECTION('center_axis',(0.,1.,0.));
#27470=DIRECTION('ref_axis',(1.,0.,0.));
#27471=DIRECTION('center_axis',(0.,1.,0.));
#27472=DIRECTION('ref_axis',(-7.6571373978539E-16,0.,-1.));
#27473=DIRECTION('center_axis',(0.,1.,0.));
#27474=DIRECTION('ref_axis',(1.,0.,0.));
#27475=DIRECTION('center_axis',(0.,1.,0.));
#27476=DIRECTION('ref_axis',(1.,0.,0.));
#27477=DIRECTION('center_axis',(0.,1.,0.));
#27478=DIRECTION('ref_axis',(0.,0.,1.));
#27479=DIRECTION('',(-1.04972719113862E-16,0.515038074910055,-0.857167300702112));
#27480=DIRECTION('center_axis',(0.,-1.,0.));
#27481=DIRECTION('ref_axis',(0.,0.,-1.));
#27482=DIRECTION('center_axis',(0.,0.,1.));
#27483=DIRECTION('ref_axis',(0.819152044288992,0.573576436351046,0.));
#27484=DIRECTION('center_axis',(0.,0.,-1.));
#27485=DIRECTION('ref_axis',(0.819152044288992,0.573576436351046,0.));
#27486=DIRECTION('',(0.,0.,1.));
#27487=DIRECTION('',(0.,0.,1.));
#27488=DIRECTION('center_axis',(0.,0.,-1.));
#27489=DIRECTION('ref_axis',(0.819152044288992,0.573576436351046,0.));
#27490=DIRECTION('center_axis',(0.,0.,1.));
#27491=DIRECTION('ref_axis',(1.,0.,0.));
#27492=DIRECTION('center_axis',(0.,0.,1.));
#27493=DIRECTION('ref_axis',(0.819152044288992,0.573576436351046,0.));
#27494=DIRECTION('center_axis',(0.,0.,1.));
#27495=DIRECTION('ref_axis',(-0.819152044288992,-0.573576436351046,0.));
#27496=DIRECTION('center_axis',(0.,0.,1.));
#27497=DIRECTION('ref_axis',(-0.819152044288991,0.573576436351046,0.));
#27498=DIRECTION('',(0.,0.,1.));
#27499=DIRECTION('center_axis',(0.,0.,1.));
#27500=DIRECTION('ref_axis',(-0.819152044288991,0.573576436351046,0.));
#27501=DIRECTION('center_axis',(0.,0.,1.));
#27502=DIRECTION('ref_axis',(0.819152044288992,0.573576436351046,0.));
#27503=DIRECTION('center_axis',(0.,0.,1.));
#27504=DIRECTION('ref_axis',(0.819152044288992,0.573576436351046,0.));
#27505=DIRECTION('',(0.,0.,1.));
#27506=DIRECTION('center_axis',(0.,0.,1.));
#27507=DIRECTION('ref_axis',(-0.819152044288992,-0.573576436351046,0.));
#27508=DIRECTION('center_axis',(0.,0.,1.));
#27509=DIRECTION('ref_axis',(1.,0.,0.));
#27510=DIRECTION('center_axis',(0.,0.,1.));
#27511=DIRECTION('ref_axis',(0.819152044288992,-0.573576436351046,0.));
#27512=DIRECTION('',(0.,0.,1.));
#27513=DIRECTION('center_axis',(0.,0.,1.));
#27514=DIRECTION('ref_axis',(0.819152044288992,-0.573576436351046,0.));
#27515=DIRECTION('center_axis',(0.,0.,1.));
#27516=DIRECTION('ref_axis',(-0.819152044288992,-0.573576436351046,0.));
#27517=DIRECTION('center_axis',(0.,0.,1.));
#27518=DIRECTION('ref_axis',(-0.819152044288992,-0.573576436351046,0.));
#27519=DIRECTION('',(0.,0.,1.));
#27520=DIRECTION('center_axis',(0.,0.,1.));
#27521=DIRECTION('ref_axis',(0.819152044288991,0.573576436351047,0.));
#27522=DIRECTION('center_axis',(0.,0.,1.));
#27523=DIRECTION('ref_axis',(1.,0.,0.));
#27524=DIRECTION('center_axis',(0.,0.,-1.));
#27525=DIRECTION('ref_axis',(-1.,0.,0.));
#27526=DIRECTION('',(-0.707106781186547,8.65956056235493E-17,0.707106781186547));
#27527=DIRECTION('center_axis',(0.,0.,1.));
#27528=DIRECTION('ref_axis',(-1.,0.,0.));
#27529=DIRECTION('center_axis',(0.,0.,1.));
#27530=DIRECTION('ref_axis',(-1.,0.,0.));
#27531=DIRECTION('center_axis',(0.,0.,1.));
#27532=DIRECTION('ref_axis',(1.,0.,0.));
#27533=DIRECTION('center_axis',(0.,0.,-1.));
#27534=DIRECTION('ref_axis',(-1.,0.,0.));
#27535=DIRECTION('center_axis',(0.,0.,-1.));
#27536=DIRECTION('ref_axis',(-1.,0.,0.));
#27537=DIRECTION('',(0.,0.,-1.));
#27538=DIRECTION('center_axis',(0.,0.,1.));
#27539=DIRECTION('ref_axis',(-1.,0.,0.));
#27540=DIRECTION('',(0.707106781186549,-8.65956056235495E-17,0.707106781186546));
#27541=DIRECTION('center_axis',(0.,0.,1.));
#27542=DIRECTION('ref_axis',(1.,0.,0.));
#27543=DIRECTION('center_axis',(0.,0.,1.));
#27544=DIRECTION('ref_axis',(1.,0.,0.));
#27545=DIRECTION('center_axis',(0.,0.,1.));
#27546=DIRECTION('ref_axis',(1.,0.,0.));
#27547=DIRECTION('center_axis',(0.,0.,1.));
#27548=DIRECTION('ref_axis',(1.,0.,0.));
#27549=DIRECTION('center_axis',(0.,0.,-1.));
#27550=DIRECTION('ref_axis',(1.,0.,0.));
#42776=CARTESIAN_POINT('',(0.,0.,0.));
#42777=CARTESIAN_POINT('Origin',(6.,0.,2.385));
#42778=CARTESIAN_POINT('',(5.52,-5.8783046359073E-17,2.4));
#42779=CARTESIAN_POINT('Origin',(6.,0.,2.4));
#42780=CARTESIAN_POINT('',(5.55,5.51091059616309E-17,2.37));
#42781=CARTESIAN_POINT('',(5.535,-5.6946076160352E-17,2.385));
#42782=CARTESIAN_POINT('Origin',(6.,0.,2.37));
#42783=CARTESIAN_POINT('Origin',(6.,0.,1.21));
#42784=CARTESIAN_POINT('',(5.55,-5.51091059616309E-17,0.03));
#42785=CARTESIAN_POINT('Origin',(6.,0.,0.03));
#42786=CARTESIAN_POINT('',(5.55,-5.51091059616309E-17,1.21));
#42787=CARTESIAN_POINT('Origin',(1.5,0.,2.4));
#42788=CARTESIAN_POINT('',(-1.17046999107197,-6.8,2.4));
#42789=CARTESIAN_POINT('',(1.17046999107197,-6.8,2.4));
#42790=CARTESIAN_POINT('',(0.75,-6.8,2.4));
#42791=CARTESIAN_POINT('',(1.17046999107197,6.8,2.4));
#42792=CARTESIAN_POINT('Origin',(0.,0.,2.4));
#42793=CARTESIAN_POINT('',(-1.17046999107197,6.8,2.4));
#42794=CARTESIAN_POINT('',(0.75,6.8,2.4));
#42795=CARTESIAN_POINT('Origin',(0.,0.,2.4));
#42796=CARTESIAN_POINT('',(2.52,5.19615242270663,2.4));
#42797=CARTESIAN_POINT('Origin',(3.,5.19615242270663,2.4));
#42798=CARTESIAN_POINT('',(-6.48,6.76005033129339E-16,2.4));
#42799=CARTESIAN_POINT('Origin',(-6.,7.34788079488412E-16,2.4));
#42800=CARTESIAN_POINT('',(2.52,-5.19615242270663,2.4));
#42801=CARTESIAN_POINT('Origin',(3.,-5.19615242270663,2.4));
#42802=CARTESIAN_POINT('',(1.55,1.8982025386784E-16,2.4));
#42803=CARTESIAN_POINT('Origin',(0.,0.,2.4));
#42804=CARTESIAN_POINT('',(-0.3,4.8,2.4));
#42805=CARTESIAN_POINT('Origin',(0.,4.8,2.4));
#42806=CARTESIAN_POINT('',(-3.48,-5.19615242270663,2.4));
#42807=CARTESIAN_POINT('Origin',(-3.,-5.19615242270663,2.4));
#42808=CARTESIAN_POINT('',(-3.48,5.19615242270663,2.4));
#42809=CARTESIAN_POINT('Origin',(-3.,5.19615242270663,2.4));
#42810=CARTESIAN_POINT('Origin',(6.,0.,0.015));
#42811=CARTESIAN_POINT('',(5.52,5.8783046359073E-17,0.));
#42812=CARTESIAN_POINT('Origin',(6.,0.,0.));
#42813=CARTESIAN_POINT('',(5.535,5.6946076160352E-17,0.015));
#42814=CARTESIAN_POINT('Origin',(6.9,0.,0.));
#42815=CARTESIAN_POINT('',(1.17046999107197,-6.8,0.));
#42816=CARTESIAN_POINT('',(-1.17046999107197,-6.8,0.));
#42817=CARTESIAN_POINT('',(3.45,-6.8,0.));
#42818=CARTESIAN_POINT('',(-1.17046999107197,6.8,0.));
#42819=CARTESIAN_POINT('Origin',(0.,0.,0.));
#42820=CARTESIAN_POINT('',(1.17046999107197,6.8,0.));
#42821=CARTESIAN_POINT('',(3.45,6.8,0.));
#42822=CARTESIAN_POINT('Origin',(0.,0.,0.));
#42823=CARTESIAN_POINT('',(2.52,5.19615242270663,0.));
#42824=CARTESIAN_POINT('Origin',(3.,5.19615242270663,0.));
#42825=CARTESIAN_POINT('',(-6.48,7.93571125847485E-16,0.));
#42826=CARTESIAN_POINT('Origin',(-6.,7.34788079488412E-16,0.));
#42827=CARTESIAN_POINT('',(2.52,-5.19615242270663,0.));
#42828=CARTESIAN_POINT('Origin',(3.,-5.19615242270663,0.));
#42829=CARTESIAN_POINT('',(-1.84309209965023,1.29054698178985,0.));
#42830=CARTESIAN_POINT('',(1.84309209965023,1.29054698178985,0.));
#42831=CARTESIAN_POINT('Origin',(-2.22044604925031E-16,-4.44089209850063E-16,
0.));
#42832=CARTESIAN_POINT('',(2.41649853065253,1.69205048723559,0.));
#42833=CARTESIAN_POINT('Origin',(2.12979531515138,1.49129873451272,0.));
#42834=CARTESIAN_POINT('',(-2.41649853065253,1.69205048723559,0.));
#42835=CARTESIAN_POINT('Origin',(0.,8.88178419700125E-16,0.));
#42836=CARTESIAN_POINT('Origin',(-2.12979531515138,1.49129873451272,0.));
#42837=CARTESIAN_POINT('',(1.84309209965023,-1.29054698178985,0.));
#42838=CARTESIAN_POINT('',(-1.84309209965023,-1.29054698178985,0.));
#42839=CARTESIAN_POINT('Origin',(0.,0.,0.));
#42840=CARTESIAN_POINT('',(-2.41649853065253,-1.69205048723559,0.));
#42841=CARTESIAN_POINT('Origin',(-2.12979531515138,-1.49129873451272,0.));
#42842=CARTESIAN_POINT('',(2.41649853065253,-1.69205048723559,0.));
#42843=CARTESIAN_POINT('Origin',(0.,0.,0.));
#42844=CARTESIAN_POINT('Origin',(2.12979531515138,-1.49129873451272,0.));
#42845=CARTESIAN_POINT('',(1.55,-1.8982025386784E-16,0.));
#42846=CARTESIAN_POINT('Origin',(0.,0.,0.));
#42847=CARTESIAN_POINT('',(-3.48,-5.19615242270663,0.));
#42848=CARTESIAN_POINT('Origin',(-3.,-5.19615242270663,0.));
#42849=CARTESIAN_POINT('',(-3.48,5.19615242270663,0.));
#42850=CARTESIAN_POINT('Origin',(-3.,5.19615242270663,0.));
#42851=CARTESIAN_POINT('Origin',(3.,5.19615242270663,2.385));
#42852=CARTESIAN_POINT('',(2.55,5.19615242270663,2.37));
#42853=CARTESIAN_POINT('',(2.535,5.19615242270663,2.385));
#42854=CARTESIAN_POINT('Origin',(3.,5.19615242270663,2.37));
#42855=CARTESIAN_POINT('Origin',(3.,5.19615242270663,1.21));
#42856=CARTESIAN_POINT('',(2.55,5.19615242270663,0.03));
#42857=CARTESIAN_POINT('Origin',(3.,5.19615242270663,0.03));
#42858=CARTESIAN_POINT('',(2.55,5.19615242270663,1.21));
#42859=CARTESIAN_POINT('Origin',(3.,5.19615242270663,0.015));
#42860=CARTESIAN_POINT('',(2.535,5.19615242270663,0.015));
#42861=CARTESIAN_POINT('Origin',(-3.,5.19615242270663,2.385));
#42862=CARTESIAN_POINT('',(-3.45,5.19615242270663,2.37));
#42863=CARTESIAN_POINT('',(-3.465,5.19615242270663,2.385));
#42864=CARTESIAN_POINT('Origin',(-3.,5.19615242270663,2.37));
#42865=CARTESIAN_POINT('Origin',(-3.,5.19615242270663,1.21));
#42866=CARTESIAN_POINT('',(-3.45,5.19615242270663,0.03));
#42867=CARTESIAN_POINT('Origin',(-3.,5.19615242270663,0.03));
#42868=CARTESIAN_POINT('',(-3.45,5.19615242270663,1.21));
#42869=CARTESIAN_POINT('Origin',(-3.,5.19615242270663,0.015));
#42870=CARTESIAN_POINT('',(-3.465,5.19615242270663,0.015));
#42871=CARTESIAN_POINT('Origin',(-6.,7.34788079488412E-16,2.385));
#42872=CARTESIAN_POINT('',(-6.45,7.89897185450043E-16,2.37));
#42873=CARTESIAN_POINT('',(-6.465,6.7784200332806E-16,2.385));
#42874=CARTESIAN_POINT('Origin',(-6.,7.34788079488412E-16,2.37));
#42875=CARTESIAN_POINT('Origin',(-6.,7.34788079488412E-16,1.21));
#42876=CARTESIAN_POINT('',(-6.45,6.79678973526781E-16,0.03));
#42877=CARTESIAN_POINT('Origin',(-6.,7.34788079488412E-16,0.03));
#42878=CARTESIAN_POINT('',(-6.45,6.79678973526781E-16,1.21));
#42879=CARTESIAN_POINT('Origin',(-6.,7.34788079488412E-16,0.015));
#42880=CARTESIAN_POINT('',(-6.465,7.91734155648764E-16,0.015));
#42881=CARTESIAN_POINT('Origin',(-3.,-5.19615242270663,2.385));
#42882=CARTESIAN_POINT('',(-3.45,-5.19615242270663,2.37));
#42883=CARTESIAN_POINT('',(-3.465,-5.19615242270663,2.385));
#42884=CARTESIAN_POINT('Origin',(-3.,-5.19615242270663,2.37));
#42885=CARTESIAN_POINT('Origin',(-3.,-5.19615242270663,1.21));
#42886=CARTESIAN_POINT('',(-3.45,-5.19615242270663,0.03));
#42887=CARTESIAN_POINT('Origin',(-3.,-5.19615242270663,0.03));
#42888=CARTESIAN_POINT('',(-3.45,-5.19615242270663,1.21));
#42889=CARTESIAN_POINT('Origin',(-3.,-5.19615242270663,0.015));
#42890=CARTESIAN_POINT('',(-3.465,-5.19615242270663,0.015));
#42891=CARTESIAN_POINT('Origin',(3.,-5.19615242270663,2.385));
#42892=CARTESIAN_POINT('',(2.55,-5.19615242270663,2.37));
#42893=CARTESIAN_POINT('',(2.535,-5.19615242270663,2.385));
#42894=CARTESIAN_POINT('Origin',(3.,-5.19615242270663,2.37));
#42895=CARTESIAN_POINT('Origin',(3.,-5.19615242270663,1.21));
#42896=CARTESIAN_POINT('',(2.55,-5.19615242270663,0.03));
#42897=CARTESIAN_POINT('Origin',(3.,-5.19615242270663,0.03));
#42898=CARTESIAN_POINT('',(2.55,-5.19615242270663,1.21));
#42899=CARTESIAN_POINT('Origin',(3.,-5.19615242270663,0.015));
#42900=CARTESIAN_POINT('',(2.535,-5.19615242270663,0.015));
#42901=CARTESIAN_POINT('Origin',(0.,4.8,1.715));
#42902=CARTESIAN_POINT('',(0.3,4.8,1.71961524227066));
#42903=CARTESIAN_POINT('',(-0.3,4.8,1.71961524227066));
#42904=CARTESIAN_POINT('Ctrl Pts',(0.3,4.8,1.71961524227066));
#42905=CARTESIAN_POINT('Ctrl Pts',(0.3,4.83849152008815,1.71961524227066));
#42906=CARTESIAN_POINT('Ctrl Pts',(0.292165675343028,4.87894158037899,1.72434763078588));
#42907=CARTESIAN_POINT('Ctrl Pts',(0.261368612920868,4.95257470785234,1.7403588037382));
#42908=CARTESIAN_POINT('Ctrl Pts',(0.23842674843931,4.98583732027262,1.75131014026465));
#42909=CARTESIAN_POINT('Ctrl Pts',(0.185909000941879,5.03835506777005,1.77115998302115));
#42910=CARTESIAN_POINT('Ctrl Pts',(0.152622227434313,5.06134952397737,1.78147945231184));
#42911=CARTESIAN_POINT('Ctrl Pts',(0.0788835226466574,5.09218917176074,
1.7959775905052));
#42912=CARTESIAN_POINT('Ctrl Pts',(0.0383865903326067,5.1,1.8));
#42913=CARTESIAN_POINT('Ctrl Pts',(-0.0383865903326067,5.1,1.8));
#42914=CARTESIAN_POINT('Ctrl Pts',(-0.078883522646657,5.09218917176074,
1.7959775905052));
#42915=CARTESIAN_POINT('Ctrl Pts',(-0.152622227434313,5.06134952397737,
1.78147945231184));
#42916=CARTESIAN_POINT('Ctrl Pts',(-0.185909000941879,5.03835506777005,
1.77115998302115));
#42917=CARTESIAN_POINT('Ctrl Pts',(-0.23842674843931,4.98583732027262,1.75131014026465));
#42918=CARTESIAN_POINT('Ctrl Pts',(-0.261368612920868,4.95257470785235,
1.7403588037382));
#42919=CARTESIAN_POINT('Ctrl Pts',(-0.292165675343028,4.87894158037899,
1.72434763078588));
#42920=CARTESIAN_POINT('Ctrl Pts',(-0.3,4.83849152008815,1.71961524227066));
#42921=CARTESIAN_POINT('Ctrl Pts',(-0.3,4.8,1.71961524227066));
#42922=CARTESIAN_POINT('Ctrl Pts',(-0.3,4.8,1.71961524227066));
#42923=CARTESIAN_POINT('Ctrl Pts',(-0.3,4.76150847991185,1.71961524227066));
#42924=CARTESIAN_POINT('Ctrl Pts',(-0.292165675343028,4.72105841962101,
1.72434763078588));
#42925=CARTESIAN_POINT('Ctrl Pts',(-0.261368612920868,4.64742529214765,
1.7403588037382));
#42926=CARTESIAN_POINT('Ctrl Pts',(-0.23842674843931,4.61416267972738,1.75131014026465));
#42927=CARTESIAN_POINT('Ctrl Pts',(-0.185909000941879,4.56164493222995,
1.77115998302115));
#42928=CARTESIAN_POINT('Ctrl Pts',(-0.152622227434313,4.53865047602263,
1.78147945231184));
#42929=CARTESIAN_POINT('Ctrl Pts',(-0.0788835226466568,4.50781082823926,
1.7959775905052));
#42930=CARTESIAN_POINT('Ctrl Pts',(-0.0383865903326067,4.5,1.8));
#42931=CARTESIAN_POINT('Ctrl Pts',(0.0383865903326067,4.5,1.8));
#42932=CARTESIAN_POINT('Ctrl Pts',(0.0788835226466565,4.50781082823926,
1.7959775905052));
#42933=CARTESIAN_POINT('Ctrl Pts',(0.152622227434312,4.53865047602263,1.78147945231184));
#42934=CARTESIAN_POINT('Ctrl Pts',(0.185909000941879,4.56164493222995,1.77115998302115));
#42935=CARTESIAN_POINT('Ctrl Pts',(0.23842674843931,4.61416267972738,1.75131014026465));
#42936=CARTESIAN_POINT('Ctrl Pts',(0.261368612920868,4.64742529214765,1.7403588037382));
#42937=CARTESIAN_POINT('Ctrl Pts',(0.292165675343028,4.72105841962101,1.72434763078588));
#42938=CARTESIAN_POINT('Ctrl Pts',(0.3,4.76150847991185,1.71961524227066));
#42939=CARTESIAN_POINT('Ctrl Pts',(0.3,4.8,1.71961524227066));
#42940=CARTESIAN_POINT('',(-0.3,4.8,1.715));
#42941=CARTESIAN_POINT('Origin',(0.,6.76,1.2));
#42942=CARTESIAN_POINT('',(-1.12434822629719E-16,6.8,0.2819));
#42943=CARTESIAN_POINT('Origin',(0.,6.8,1.2));
#42944=CARTESIAN_POINT('',(1.0263764823654E-16,6.72,0.3619));
#42945=CARTESIAN_POINT('',(-1.07536235433129E-16,6.76,0.3219));
#42946=CARTESIAN_POINT('Origin',(0.,6.72,1.2));
#42947=CARTESIAN_POINT('Origin',(0.,6.115,1.2));
#42948=CARTESIAN_POINT('',(-1.0263764823654E-16,5.4,0.3619));
#42949=CARTESIAN_POINT('Origin',(0.,5.4,1.2));
#42950=CARTESIAN_POINT('',(-1.0263764823654E-16,6.115,0.3619));
#42951=CARTESIAN_POINT('Origin',(0.,6.8,1.2));
#42952=CARTESIAN_POINT('',(1.66132477258362,6.8,2.3));
#42953=CARTESIAN_POINT('Ctrl Pts',(1.66132477258361,6.8,2.3));
#42954=CARTESIAN_POINT('Ctrl Pts',(1.41413171714607,6.8,2.35866684951557));
#42955=CARTESIAN_POINT('Ctrl Pts',(1.17046999107197,6.8,2.4));
#42956=CARTESIAN_POINT('',(1.66132477258362,6.8,0.1));
#42957=CARTESIAN_POINT('',(1.66132477258362,6.8,1.2));
#42958=CARTESIAN_POINT('Ctrl Pts',(1.17046999107197,6.8,-1.11022302462516E-16));
#42959=CARTESIAN_POINT('Ctrl Pts',(1.4141317171461,6.8,0.0413331504844302));
#42960=CARTESIAN_POINT('Ctrl Pts',(1.66132477258362,6.8,0.1));
#42961=CARTESIAN_POINT('',(-1.66132477258362,6.8,0.1));
#42962=CARTESIAN_POINT('Ctrl Pts',(-1.66132477258362,6.8,0.1));
#42963=CARTESIAN_POINT('Ctrl Pts',(-1.4141317171461,6.8,0.0413331504844302));
#42964=CARTESIAN_POINT('Ctrl Pts',(-1.17046999107197,6.8,-1.11022302462516E-16));
#42965=CARTESIAN_POINT('',(-1.66132477258362,6.8,2.3));
#42966=CARTESIAN_POINT('',(-1.66132477258362,6.8,1.2));
#42967=CARTESIAN_POINT('Ctrl Pts',(-1.17046999107197,6.8,2.4));
#42968=CARTESIAN_POINT('Ctrl Pts',(-1.41413171714607,6.8,2.35866684951557));
#42969=CARTESIAN_POINT('Ctrl Pts',(-1.66132477258361,6.8,2.3));
#42970=CARTESIAN_POINT('Origin',(0.,-6.76,1.2));
#42971=CARTESIAN_POINT('',(1.12434822629719E-16,-6.8,0.2819));
#42972=CARTESIAN_POINT('Origin',(0.,-6.8,1.2));
#42973=CARTESIAN_POINT('',(-1.0263764823654E-16,-6.72,0.3619));
#42974=CARTESIAN_POINT('',(1.07536235433129E-16,-6.76,0.3219));
#42975=CARTESIAN_POINT('Origin',(0.,-6.72,1.2));
#42976=CARTESIAN_POINT('Origin',(0.,-6.115,1.2));
#42977=CARTESIAN_POINT('',(-1.0263764823654E-16,-5.4,0.3619));
#42978=CARTESIAN_POINT('',(-1.0263764823654E-16,-6.115,0.3619));
#42979=CARTESIAN_POINT('Origin',(0.,-5.4,1.2));
#42980=CARTESIAN_POINT('Origin',(0.,-6.8,1.2));
#42981=CARTESIAN_POINT('',(-1.66132477258362,-6.8,2.3));
#42982=CARTESIAN_POINT('Ctrl Pts',(-1.66132477258361,-6.8,2.3));
#42983=CARTESIAN_POINT('Ctrl Pts',(-1.41413171714607,-6.8,2.35866684951557));
#42984=CARTESIAN_POINT('Ctrl Pts',(-1.17046999107197,-6.8,2.4));
#42985=CARTESIAN_POINT('',(-1.66132477258362,-6.8,0.1));
#42986=CARTESIAN_POINT('',(-1.66132477258362,-6.8,1.2));
#42987=CARTESIAN_POINT('Ctrl Pts',(-1.17046999107197,-6.8,-1.52655665885959E-16));
#42988=CARTESIAN_POINT('Ctrl Pts',(-1.4141317171461,-6.8,0.04133315048443));
#42989=CARTESIAN_POINT('Ctrl Pts',(-1.66132477258362,-6.8,0.1));
#42990=CARTESIAN_POINT('',(1.66132477258362,-6.8,0.1));
#42991=CARTESIAN_POINT('Ctrl Pts',(1.66132477258362,-6.8,0.1));
#42992=CARTESIAN_POINT('Ctrl Pts',(1.4141317171461,-6.8,0.04133315048443));
#42993=CARTESIAN_POINT('Ctrl Pts',(1.17046999107197,-6.8,-1.52655665885959E-16));
#42994=CARTESIAN_POINT('',(1.66132477258362,-6.8,2.3));
#42995=CARTESIAN_POINT('',(1.66132477258362,-6.8,1.2));
#42996=CARTESIAN_POINT('Ctrl Pts',(1.17046999107197,-6.8,2.4));
#42997=CARTESIAN_POINT('Ctrl Pts',(1.41413171714607,-6.8,2.35866684951557));
#42998=CARTESIAN_POINT('Ctrl Pts',(1.66132477258361,-6.8,2.3));
#42999=CARTESIAN_POINT('Origin',(0.,-3.8,1.2));
#43000=CARTESIAN_POINT('',(-7.34788079488412E-17,-5.4,0.6));
#43001=CARTESIAN_POINT('Origin',(0.,-5.4,1.2));
#43002=CARTESIAN_POINT('',(-5.75560856861423E-17,-2.95,0.6));
#43003=CARTESIAN_POINT('',(-7.34788079488412E-17,-3.8,0.6));
#43004=CARTESIAN_POINT('',(-0.565685424949239,-2.89525473836069,1.));
#43005=CARTESIAN_POINT('Ctrl Pts',(-0.565685424949238,-2.89525473836069,
1.));
#43006=CARTESIAN_POINT('Ctrl Pts',(-0.562127356844792,-2.89594992667728,
0.98993626366169));
#43007=CARTESIAN_POINT('Ctrl Pts',(-0.558298097879191,-2.89669131763276,
0.979960768047715));
#43008=CARTESIAN_POINT('Ctrl Pts',(-0.523558121743437,-2.90333610967591,
0.896216130064144));
#43009=CARTESIAN_POINT('Ctrl Pts',(-0.477417986945562,-2.91160730139143,
0.828889849521705));
#43010=CARTESIAN_POINT('Ctrl Pts',(-0.371113340250497,-2.92705646583967,
0.722585202826639));
#43011=CARTESIAN_POINT('Ctrl Pts',(-0.303785706689727,-2.93525235179074,
0.676442570241645));
#43012=CARTESIAN_POINT('Ctrl Pts',(-0.156018762471502,-2.94680339855193,
0.615144217035157));
#43013=CARTESIAN_POINT('Ctrl Pts',(-0.0755623283236566,-2.95,0.6));
#43014=CARTESIAN_POINT('Ctrl Pts',(-1.38777878078145E-17,-2.95,0.6));
#43015=CARTESIAN_POINT('',(-0.565685424949238,-2.2,1.));
#43016=CARTESIAN_POINT('',(-0.565685424949238,-3.8,1.));
#43017=CARTESIAN_POINT('',(0.565685424949238,-2.2,1.));
#43018=CARTESIAN_POINT('Origin',(0.,-2.2,1.2));
#43019=CARTESIAN_POINT('',(0.565685424949239,-2.89525473836069,1.));
#43020=CARTESIAN_POINT('',(0.565685424949238,-3.8,1.));
#43021=CARTESIAN_POINT('Ctrl Pts',(-1.38777878078145E-17,-2.95,0.6));
#43022=CARTESIAN_POINT('Ctrl Pts',(0.0755623283236566,-2.95,0.6));
#43023=CARTESIAN_POINT('Ctrl Pts',(0.156018762471502,-2.94680339855193,
0.615144217035157));
#43024=CARTESIAN_POINT('Ctrl Pts',(0.303785706689727,-2.93525235179075,
0.676442570241645));
#43025=CARTESIAN_POINT('Ctrl Pts',(0.371113340250496,-2.92705646583967,
0.722585202826639));
#43026=CARTESIAN_POINT('Ctrl Pts',(0.477417986945562,-2.91160730139143,
0.828889849521705));
#43027=CARTESIAN_POINT('Ctrl Pts',(0.523558121743436,-2.90333610967591,
0.896216130064144));
#43028=CARTESIAN_POINT('Ctrl Pts',(0.55829809787919,-2.89669131763276,0.979960768047715));
#43029=CARTESIAN_POINT('Ctrl Pts',(0.562127356844792,-2.89594992667728,
0.98993626366169));
#43030=CARTESIAN_POINT('Ctrl Pts',(0.565685424949238,-2.89525473836069,
1.));
#43031=CARTESIAN_POINT('Origin',(0.,-3.8,1.2));
#43032=CARTESIAN_POINT('',(0.47169905660283,-2.2,0.829190075645216));
#43033=CARTESIAN_POINT('',(-0.47169905660283,-2.2,0.829190075645216));
#43034=CARTESIAN_POINT('Ctrl Pts',(0.47169905660283,-2.2,0.829190075645216));
#43035=CARTESIAN_POINT('Ctrl Pts',(0.456732221663335,-2.20320901905513,
0.810151097835833));
#43036=CARTESIAN_POINT('Ctrl Pts',(0.44080709474806,-2.20646161675427,0.792278957324203));
#43037=CARTESIAN_POINT('Ctrl Pts',(0.371203803057213,-2.21982587642206,
0.722675665633356));
#43038=CARTESIAN_POINT('Ctrl Pts',(0.303979231951913,-2.2306075153835,0.676556496463189));
#43039=CARTESIAN_POINT('Ctrl Pts',(0.156255272557804,-2.24579552733492,
0.615208780719168));
#43040=CARTESIAN_POINT('Ctrl Pts',(0.0757269887719169,-2.25,0.6));
#43041=CARTESIAN_POINT('Ctrl Pts',(-0.0757269887719168,-2.25,0.6));
#43042=CARTESIAN_POINT('Ctrl Pts',(-0.156255272557804,-2.24579552733492,
0.615208780719168));
#43043=CARTESIAN_POINT('Ctrl Pts',(-0.303979231951912,-2.2306075153835,
0.676556496463189));
#43044=CARTESIAN_POINT('Ctrl Pts',(-0.371203803057213,-2.21982587642206,
0.722675665633356));
#43045=CARTESIAN_POINT('Ctrl Pts',(-0.44080709474806,-2.20646161675427,
0.792278957324203));
#43046=CARTESIAN_POINT('Ctrl Pts',(-0.456732221663335,-2.20320901905513,
0.810151097835833));
#43047=CARTESIAN_POINT('Ctrl Pts',(-0.47169905660283,-2.2,0.829190075645216));
#43048=CARTESIAN_POINT('',(-7.34788079488412E-17,-2.2,0.6));
#43049=CARTESIAN_POINT('Origin',(0.,-2.2,1.2));
#43050=CARTESIAN_POINT('Origin',(0.,-2.2,1.2));
#43051=CARTESIAN_POINT('Origin',(0.,-5.4,1.8));
#43052=CARTESIAN_POINT('Origin',(0.,-2.2,1.2));
#43053=CARTESIAN_POINT('',(0.538458996921356,-2.18461939674499,1.));
#43054=CARTESIAN_POINT('Ctrl Pts',(0.538458996921356,-2.18461939674499,
1.));
#43055=CARTESIAN_POINT('Ctrl Pts',(0.535129652878092,-2.18544000433303,
0.987114058586867));
#43056=CARTESIAN_POINT('Ctrl Pts',(0.531468422935026,-2.18633440357531,
0.974298290302466));
#43057=CARTESIAN_POINT('Ctrl Pts',(0.512986185718411,-2.1907915344852,0.915394770294079));
#43058=CARTESIAN_POINT('Ctrl Pts',(0.494116619449461,-2.19519348034269,
0.870650612337028));
#43059=CARTESIAN_POINT('Ctrl Pts',(0.471699056602829,-2.2,0.829190075645216));
#43060=CARTESIAN_POINT('Ctrl Pts',(0.565685424949238,-2.2,1.));
#43061=CARTESIAN_POINT('Ctrl Pts',(0.551775493286436,-2.1921200678861,1.));
#43062=CARTESIAN_POINT('Ctrl Pts',(0.538458996921356,-2.18461939674499,
1.));
#43063=CARTESIAN_POINT('',(-0.538458996921356,-2.18461939674499,1.));
#43064=CARTESIAN_POINT('Ctrl Pts',(-0.538458996921356,-2.18461939674499,
1.));
#43065=CARTESIAN_POINT('Ctrl Pts',(-0.551775493286438,-2.1921200678861,
1.));
#43066=CARTESIAN_POINT('Ctrl Pts',(-0.565685424949238,-2.2,1.));
#43067=CARTESIAN_POINT('Ctrl Pts',(-0.471699056602829,-2.2,0.829190075645216));
#43068=CARTESIAN_POINT('Ctrl Pts',(-0.494116619449461,-2.19519348034269,
0.870650612337028));
#43069=CARTESIAN_POINT('Ctrl Pts',(-0.512986185718411,-2.1907915344852,
0.915394770294079));
#43070=CARTESIAN_POINT('Ctrl Pts',(-0.531468422935026,-2.18633440357531,
0.974298290302465));
#43071=CARTESIAN_POINT('Ctrl Pts',(-0.535129652878092,-2.18544000433303,
0.987114058586867));
#43072=CARTESIAN_POINT('Ctrl Pts',(-0.538458996921356,-2.18461939674499,
1.));
#43073=CARTESIAN_POINT('',(0.,-1.83948362858346,1.2));
#43074=CARTESIAN_POINT('',(-7.34788079488412E-17,-2.2,0.6));
#43075=CARTESIAN_POINT('Origin',(0.,0.,0.));
#43076=CARTESIAN_POINT('',(-1.84309209965023,-1.29054698178985,1.));
#43077=CARTESIAN_POINT('Origin',(0.,0.,1.));
#43078=CARTESIAN_POINT('',(-1.84309209965023,-1.29054698178985,0.));
#43079=CARTESIAN_POINT('',(1.84309209965023,-1.29054698178985,1.));
#43080=CARTESIAN_POINT('',(1.84309209965023,-1.29054698178985,0.));
#43081=CARTESIAN_POINT('Origin',(0.,0.,1.));
#43082=CARTESIAN_POINT('Origin',(0.,-2.04564936725636,1.));
#43083=CARTESIAN_POINT('',(-2.41649853065253,-1.69205048723559,1.));
#43084=CARTESIAN_POINT('Origin',(0.,0.,1.));
#43085=CARTESIAN_POINT('Origin',(-2.12979531515138,-1.49129873451272,1.));
#43086=CARTESIAN_POINT('Origin',(0.,0.,0.0499999999999998));
#43087=CARTESIAN_POINT('Origin',(0.,0.,0.1));
#43088=CARTESIAN_POINT('Origin',(0.,0.,1.2));
#43089=CARTESIAN_POINT('Origin',(0.,0.,2.3));
#43090=CARTESIAN_POINT('Origin',(0.,0.,2.35));
#43091=CARTESIAN_POINT('Origin',(0.,3.8,1.2));
#43092=CARTESIAN_POINT('',(-0.565685424949238,2.89525473836069,1.));
#43093=CARTESIAN_POINT('',(-0.565685424949238,2.2,1.));
#43094=CARTESIAN_POINT('',(-0.565685424949238,3.8,1.));
#43095=CARTESIAN_POINT('',(-2.04493445488446E-18,2.95,0.6));
#43096=CARTESIAN_POINT('Ctrl Pts',(4.16333634234434E-17,2.95,0.6));
#43097=CARTESIAN_POINT('Ctrl Pts',(-0.0755623283236565,2.95,0.6));
#43098=CARTESIAN_POINT('Ctrl Pts',(-0.156018762471502,2.94680339855193,
0.615144217035157));
#43099=CARTESIAN_POINT('Ctrl Pts',(-0.303785706689727,2.93525235179075,
0.676442570241645));
#43100=CARTESIAN_POINT('Ctrl Pts',(-0.371113340250496,2.92705646583967,
0.722585202826639));
#43101=CARTESIAN_POINT('Ctrl Pts',(-0.477417986945562,2.91160730139143,
0.828889849521705));
#43102=CARTESIAN_POINT('Ctrl Pts',(-0.523558121743437,2.90333610967591,
0.896216130064144));
#43103=CARTESIAN_POINT('Ctrl Pts',(-0.558298097879191,2.89669131763276,
0.979960768047715));
#43104=CARTESIAN_POINT('Ctrl Pts',(-0.562127356844792,2.89594992667728,
0.989936263661689));
#43105=CARTESIAN_POINT('Ctrl Pts',(-0.565685424949238,2.89525473836069,
1.));
#43106=CARTESIAN_POINT('',(-7.34788079488412E-17,5.4,0.6));
#43107=CARTESIAN_POINT('',(-7.34788079488412E-17,3.8,0.6));
#43108=CARTESIAN_POINT('Origin',(0.,5.4,1.2));
#43109=CARTESIAN_POINT('',(0.565685424949238,2.89525473836069,1.));
#43110=CARTESIAN_POINT('Ctrl Pts',(0.565685424949238,2.89525473836069,1.));
#43111=CARTESIAN_POINT('Ctrl Pts',(0.562127356844792,2.89594992667728,0.98993626366169));
#43112=CARTESIAN_POINT('Ctrl Pts',(0.55829809787919,2.89669131763276,0.979960768047715));
#43113=CARTESIAN_POINT('Ctrl Pts',(0.523558121743437,2.90333610967591,0.896216130064144));
#43114=CARTESIAN_POINT('Ctrl Pts',(0.477417986945562,2.91160730139143,0.828889849521705));
#43115=CARTESIAN_POINT('Ctrl Pts',(0.371113340250497,2.92705646583967,0.722585202826639));
#43116=CARTESIAN_POINT('Ctrl Pts',(0.303785706689727,2.93525235179075,0.676442570241645));
#43117=CARTESIAN_POINT('Ctrl Pts',(0.156018762471502,2.94680339855193,0.615144217035157));
#43118=CARTESIAN_POINT('Ctrl Pts',(0.0755623283236566,2.95,0.6));
#43119=CARTESIAN_POINT('Ctrl Pts',(4.16333634234434E-17,2.95,0.6));
#43120=CARTESIAN_POINT('',(0.565685424949238,2.2,1.));
#43121=CARTESIAN_POINT('',(0.565685424949238,3.8,1.));
#43122=CARTESIAN_POINT('Origin',(0.,2.2,1.2));
#43123=CARTESIAN_POINT('Origin',(0.,3.8,1.2));
#43124=CARTESIAN_POINT('',(-0.47169905660283,2.2,0.829190075645216));
#43125=CARTESIAN_POINT('',(0.471699056602829,2.2,0.829190075645216));
#43126=CARTESIAN_POINT('Ctrl Pts',(-0.47169905660283,2.2,0.829190075645216));
#43127=CARTESIAN_POINT('Ctrl Pts',(-0.456732221663335,2.20320901905513,
0.810151097835833));
#43128=CARTESIAN_POINT('Ctrl Pts',(-0.44080709474806,2.20646161675427,0.792278957324203));
#43129=CARTESIAN_POINT('Ctrl Pts',(-0.371203803057213,2.21982587642206,
0.722675665633356));
#43130=CARTESIAN_POINT('Ctrl Pts',(-0.303979231951913,2.2306075153835,0.676556496463189));
#43131=CARTESIAN_POINT('Ctrl Pts',(-0.156255272557804,2.24579552733492,
0.615208780719168));
#43132=CARTESIAN_POINT('Ctrl Pts',(-0.0757269887719169,2.25,0.6));
#43133=CARTESIAN_POINT('Ctrl Pts',(0.0757269887719168,2.25,0.6));
#43134=CARTESIAN_POINT('Ctrl Pts',(0.156255272557804,2.24579552733492,0.615208780719168));
#43135=CARTESIAN_POINT('Ctrl Pts',(0.303979231951912,2.2306075153835,0.676556496463189));
#43136=CARTESIAN_POINT('Ctrl Pts',(0.371203803057213,2.21982587642206,0.722675665633356));
#43137=CARTESIAN_POINT('Ctrl Pts',(0.44080709474806,2.20646161675427,0.792278957324203));
#43138=CARTESIAN_POINT('Ctrl Pts',(0.456732221663335,2.20320901905513,0.810151097835833));
#43139=CARTESIAN_POINT('Ctrl Pts',(0.471699056602829,2.2,0.829190075645216));
#43140=CARTESIAN_POINT('',(-7.34788079488413E-17,2.2,0.599999999999999));
#43141=CARTESIAN_POINT('Origin',(0.,2.2,1.2));
#43142=CARTESIAN_POINT('Origin',(0.,2.2,1.2));
#43143=CARTESIAN_POINT('Origin',(0.,2.01974181429173,1.2));
#43144=CARTESIAN_POINT('',(0.,1.83948362858346,1.2));
#43145=CARTESIAN_POINT('',(-3.67394039744206E-17,2.01974181429173,0.9));
#43146=CARTESIAN_POINT('',(-0.538458996921356,2.18461939674499,1.));
#43147=CARTESIAN_POINT('Ctrl Pts',(-0.538458996921356,2.18461939674499,
1.));
#43148=CARTESIAN_POINT('Ctrl Pts',(-0.535129652878092,2.18544000433303,
0.987114058586867));
#43149=CARTESIAN_POINT('Ctrl Pts',(-0.531468422935027,2.18633440357531,
0.974298290302465));
#43150=CARTESIAN_POINT('Ctrl Pts',(-0.512986185718411,2.1907915344852,0.915394770294079));
#43151=CARTESIAN_POINT('Ctrl Pts',(-0.494116619449461,2.19519348034269,
0.870650612337029));
#43152=CARTESIAN_POINT('Ctrl Pts',(-0.47169905660283,2.2,0.829190075645216));
#43153=CARTESIAN_POINT('Ctrl Pts',(-0.565685424949238,2.2,1.));
#43154=CARTESIAN_POINT('Ctrl Pts',(-0.551775493286436,2.1921200678861,1.));
#43155=CARTESIAN_POINT('Ctrl Pts',(-0.538458996921356,2.18461939674499,
1.));
#43156=CARTESIAN_POINT('',(0.538458996921356,2.18461939674499,1.));
#43157=CARTESIAN_POINT('Ctrl Pts',(0.538458996921356,2.18461939674499,1.));
#43158=CARTESIAN_POINT('Ctrl Pts',(0.551775493286434,2.1921200678861,1.));
#43159=CARTESIAN_POINT('Ctrl Pts',(0.565685424949238,2.2,1.));
#43160=CARTESIAN_POINT('Ctrl Pts',(0.47169905660283,2.2,0.829190075645216));
#43161=CARTESIAN_POINT('Ctrl Pts',(0.494116619449461,2.19519348034269,0.870650612337028));
#43162=CARTESIAN_POINT('Ctrl Pts',(0.51298618571841,2.1907915344852,0.915394770294079));
#43163=CARTESIAN_POINT('Ctrl Pts',(0.531468422935026,2.18633440357531,0.974298290302465));
#43164=CARTESIAN_POINT('Ctrl Pts',(0.535129652878092,2.18544000433303,0.987114058586867));
#43165=CARTESIAN_POINT('Ctrl Pts',(0.538458996921356,2.18461939674499,1.));
#43166=CARTESIAN_POINT('Origin',(0.,5.4,2.0381));
#43167=CARTESIAN_POINT('Origin',(-2.22044604925031E-16,-4.44089209850063E-16,
0.));
#43168=CARTESIAN_POINT('',(1.84309209965023,1.29054698178985,1.));
#43169=CARTESIAN_POINT('Origin',(-2.22044604925031E-16,-4.44089209850063E-16,
1.));
#43170=CARTESIAN_POINT('',(1.84309209965023,1.29054698178985,0.));
#43171=CARTESIAN_POINT('',(-1.84309209965023,1.29054698178985,1.));
#43172=CARTESIAN_POINT('',(-1.84309209965023,1.29054698178985,0.));
#43173=CARTESIAN_POINT('Origin',(-2.22044604925031E-16,-4.44089209850063E-16,
1.));
#43174=CARTESIAN_POINT('Origin',(-4.44089209850063E-16,2.04564936725636,
1.));
#43175=CARTESIAN_POINT('',(2.41649853065253,1.69205048723559,1.));
#43176=CARTESIAN_POINT('Origin',(0.,8.88178419700125E-16,1.));
#43177=CARTESIAN_POINT('Origin',(2.12979531515138,1.49129873451272,1.));
#43178=CARTESIAN_POINT('Origin',(-2.12979531515138,1.49129873451272,0.));
#43179=CARTESIAN_POINT('',(-2.41649853065253,1.69205048723559,1.));
#43180=CARTESIAN_POINT('',(-2.41649853065253,1.69205048723559,0.));
#43181=CARTESIAN_POINT('Origin',(-2.12979531515138,1.49129873451272,1.));
#43182=CARTESIAN_POINT('Origin',(0.,8.88178419700125E-16,0.));
#43183=CARTESIAN_POINT('Origin',(0.,8.88178419700125E-16,1.));
#43184=CARTESIAN_POINT('',(2.41649853065253,1.69205048723559,0.));
#43185=CARTESIAN_POINT('Origin',(2.12979531515138,1.49129873451272,0.));
#43186=CARTESIAN_POINT('Origin',(-4.44089209850063E-16,2.04564936725636,
1.));
#43187=CARTESIAN_POINT('Origin',(2.12979531515138,-1.49129873451272,0.));
#43188=CARTESIAN_POINT('',(2.41649853065253,-1.69205048723559,1.));
#43189=CARTESIAN_POINT('',(2.41649853065253,-1.69205048723559,0.));
#43190=CARTESIAN_POINT('Origin',(2.12979531515138,-1.49129873451272,1.));
#43191=CARTESIAN_POINT('Origin',(0.,0.,0.));
#43192=CARTESIAN_POINT('Origin',(0.,0.,1.));
#43193=CARTESIAN_POINT('',(-2.41649853065253,-1.69205048723559,0.));
#43194=CARTESIAN_POINT('Origin',(-2.12979531515138,-1.49129873451272,0.));
#43195=CARTESIAN_POINT('Origin',(0.,-2.04564936725636,1.));
#43196=CARTESIAN_POINT('Origin',(0.,0.,0.025));
#43197=CARTESIAN_POINT('',(1.5,1.83697019872103E-16,0.05));
#43198=CARTESIAN_POINT('',(1.525,-1.86758636869971E-16,0.025));
#43199=CARTESIAN_POINT('',(-1.5,-1.83697019872103E-16,0.05));
#43200=CARTESIAN_POINT('Origin',(0.,0.,0.05));
#43201=CARTESIAN_POINT('Origin',(0.,0.,0.05));
#43202=CARTESIAN_POINT('Origin',(0.,0.,1.2));
#43203=CARTESIAN_POINT('',(1.5,-1.83697019872103E-16,2.35));
#43204=CARTESIAN_POINT('',(-1.5,-1.83697019872103E-16,2.35));
#43205=CARTESIAN_POINT('Origin',(0.,0.,2.35));
#43206=CARTESIAN_POINT('Origin',(0.,0.,2.35));
#43207=CARTESIAN_POINT('',(-1.5,-1.83697019872103E-16,1.2));
#43208=CARTESIAN_POINT('Origin',(0.,0.,2.375));
#43209=CARTESIAN_POINT('',(1.525,-1.86758636869971E-16,2.375));
#43210=CARTESIAN_POINT('Origin',(0.,0.,0.0499999999999998));
#43211=CARTESIAN_POINT('Origin',(0.,0.,0.1));
#43212=CARTESIAN_POINT('Origin',(0.,0.,1.2));
#43213=CARTESIAN_POINT('Origin',(0.,0.,2.3));
#43214=CARTESIAN_POINT('Origin',(0.,0.,2.35));
#59173=UNCERTAINTY_MEASURE_WITH_UNIT(LENGTH_MEASURE(0.001),#59205,
'DISTANCE_ACCURACY_VALUE',
'Maximum model space distance between geometric entities at asserted c
onnectivities');
#59182=UNCERTAINTY_MEASURE_WITH_UNIT(LENGTH_MEASURE(0.001),#59205,
'DISTANCE_ACCURACY_VALUE',
'Maximum model space distance between geometric entities at asserted c
onnectivities');
#59195=(
GEOMETRIC_REPRESENTATION_CONTEXT(3)
GLOBAL_UNCERTAINTY_ASSIGNED_CONTEXT((#59173))
GLOBAL_UNIT_ASSIGNED_CONTEXT((#59205,#59207,#59208))
REPRESENTATION_CONTEXT('','3D')
);
#59204=(
GEOMETRIC_REPRESENTATION_CONTEXT(3)
GLOBAL_UNCERTAINTY_ASSIGNED_CONTEXT((#59182))
GLOBAL_UNIT_ASSIGNED_CONTEXT((#59205,#59207,#59208))
REPRESENTATION_CONTEXT('','3D')
);
#59205=(
LENGTH_UNIT()
NAMED_UNIT(*)
SI_UNIT(.CENTI.,.METRE.)
);
#59207=(
NAMED_UNIT(*)
PLANE_ANGLE_UNIT()
SI_UNIT($,.RADIAN.)
);
#59208=(
NAMED_UNIT(*)
SI_UNIT($,.STERADIAN.)
SOLID_ANGLE_UNIT()
);
#59221=SHAPE_DEFINITION_REPRESENTATION(#59242,#59308);
#59242=PRODUCT_DEFINITION_SHAPE('',$,#59330);
#59308=SHAPE_REPRESENTATION('',(#23866),#59195);
#59317=PRODUCT_DEFINITION_CONTEXT('part definition',#59382,'design');
#59330=PRODUCT_DEFINITION('2026-10-23-00-48-16-141',
'02_Valve_Port_Plate_D140x24_Kidney_Ports',#59351,#59317);
#59351=PRODUCT_DEFINITION_FORMATION('',$,#59396);
#59382=APPLICATION_CONTEXT(
'Core Data for Automotive Mechanical Design Process');
#59383=PRODUCT_CONTEXT('part definition',#59382,'mechanical');
#59396=PRODUCT('2026-10-23-00-48-16-141',
'02_Valve_Port_Plate_D140x24_Kidney_Ports',$,(#59383));
#59573=COLOUR_RGB('Sky Blue',0.24,0.69,0.87);
#59574=FILL_AREA_STYLE_COLOUR('',#59573);
#59575=FILL_AREA_STYLE('',(#59574));
#59576=SURFACE_STYLE_FILL_AREA(#59575);
#59577=SURFACE_SIDE_STYLE('',(#59576));
#59578=SURFACE_STYLE_USAGE(.BOTH.,#59577);
#59579=PRESENTATION_STYLE_ASSIGNMENT((#59578));
ENDSEC;
END-ISO-10303-21;
